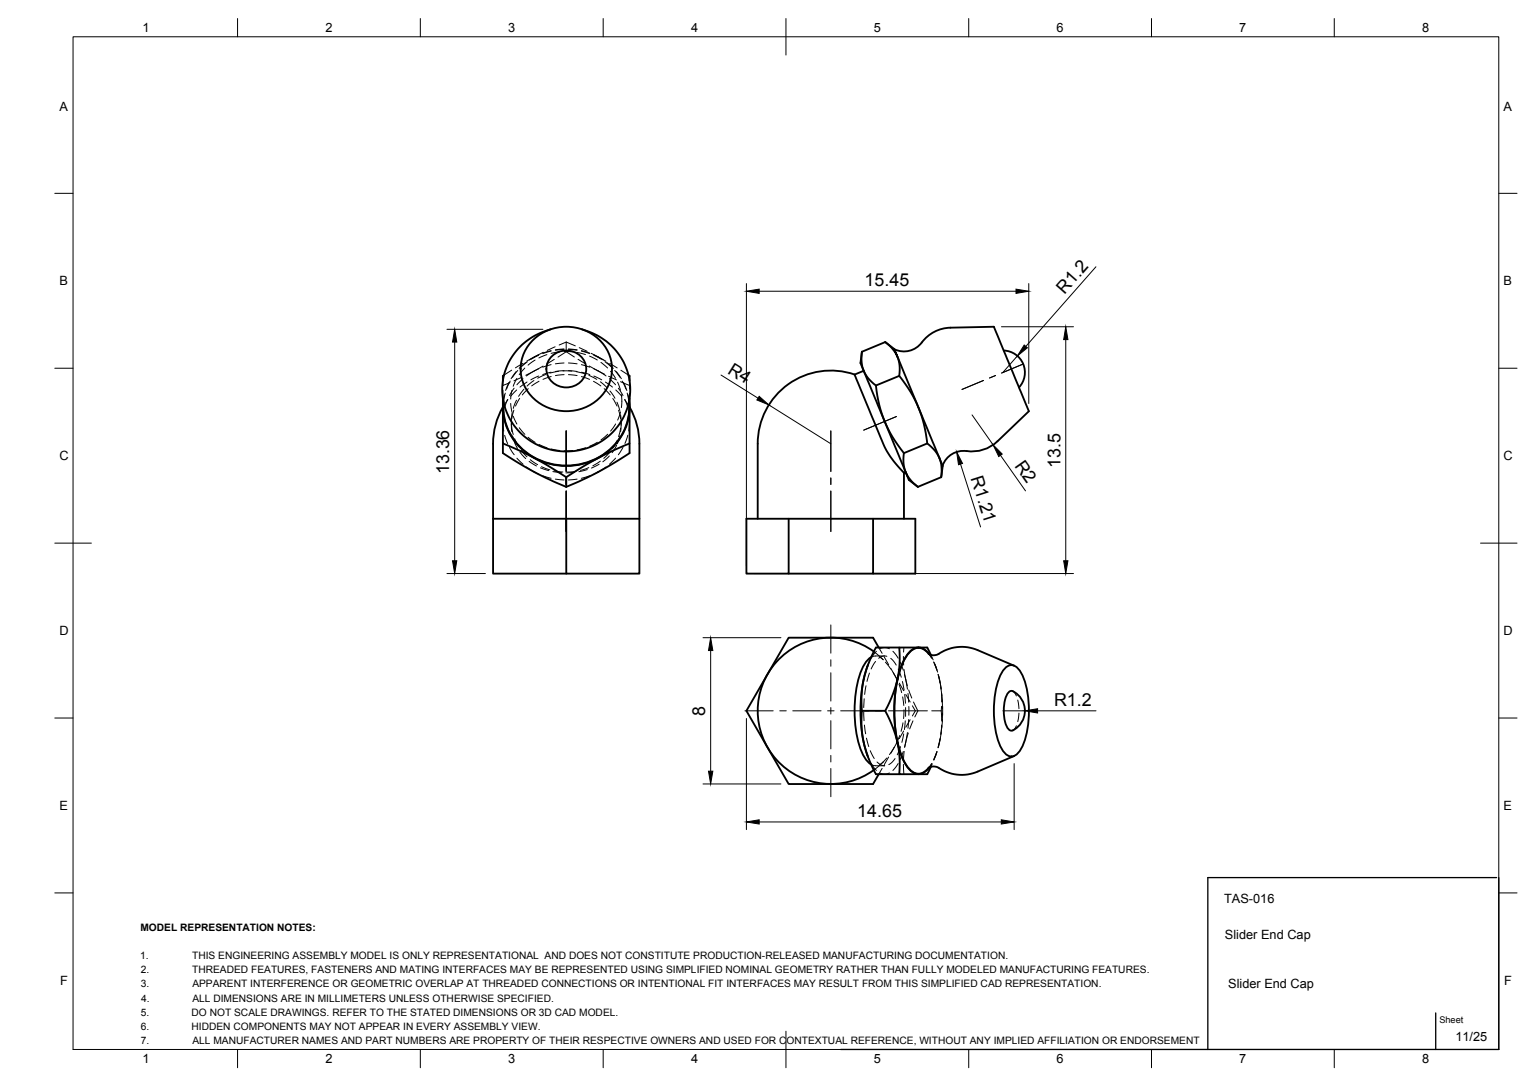
ISO-10303-21;
HEADER;
/* Generated by software containing ST-Developer
 * from STEP Tools, Inc. (www.steptools.com) 
 */

FILE_DESCRIPTION(
/* description */ ('STEP AP214'),
/* implementation_level */ '2;1');

FILE_NAME(
/* name */ 'Slider End Cap.step',
/* time_stamp */ '2026-11-15T14:55:55-08:00',
/* author */ (''),
/* organization */ (''),
/* preprocessor_version */ 'ST-DEVELOPER v20.2',
/* originating_system */ 'Autodesk Translation Framework v15.17.0.0',
/* authorisation */ '');

FILE_SCHEMA (('AUTOMOTIVE_DESIGN { 1 0 10303 214 3 1 1 }'));
ENDSEC;

DATA;
#10=MECHANICAL_DESIGN_GEOMETRIC_PRESENTATION_REPRESENTATION('',(#952),#57079);
#12=(
BOUNDED_CURVE()
B_SPLINE_CURVE(2,(#56108,#56109,#56110),.UNSPECIFIED.,.F.,.F.)
B_SPLINE_CURVE_WITH_KNOTS((3,3),(-1.38994780338837,-1.00314154055664),
 .UNSPECIFIED.)
CURVE()
GEOMETRIC_REPRESENTATION_ITEM()
RATIONAL_B_SPLINE_CURVE((1.79495951130746,1.93380011269289,1.93380011269289))
REPRESENTATION_ITEM('')
);
#13=(
BOUNDED_CURVE()
B_SPLINE_CURVE(2,(#56111,#56112,#56113),.UNSPECIFIED.,.F.,.F.)
B_SPLINE_CURVE_WITH_KNOTS((3,3),(-1.00619430729118,-0.618602381117838),
 .UNSPECIFIED.)
CURVE()
GEOMETRIC_REPRESENTATION_ITEM()
RATIONAL_B_SPLINE_CURVE((1.93745653739061,1.93745653739061,1.7983534165231))
REPRESENTATION_ITEM('')
);
#14=(
BOUNDED_CURVE()
B_SPLINE_CURVE(2,(#56119,#56120,#56121),.UNSPECIFIED.,.F.,.F.)
B_SPLINE_CURVE_WITH_KNOTS((3,3),(-1.38994780338837,-1.00314154055664),
 .UNSPECIFIED.)
CURVE()
GEOMETRIC_REPRESENTATION_ITEM()
RATIONAL_B_SPLINE_CURVE((1.79495951130745,1.93380011269288,1.93380011269288))
REPRESENTATION_ITEM('')
);
#15=(
BOUNDED_CURVE()
B_SPLINE_CURVE(2,(#56122,#56123,#56124),.UNSPECIFIED.,.F.,.F.)
B_SPLINE_CURVE_WITH_KNOTS((3,3),(-1.00619430729117,-0.618602381117832),
 .UNSPECIFIED.)
CURVE()
GEOMETRIC_REPRESENTATION_ITEM()
RATIONAL_B_SPLINE_CURVE((1.9374565373906,1.9374565373906,1.79835341652309))
REPRESENTATION_ITEM('')
);
#16=(
BOUNDED_CURVE()
B_SPLINE_CURVE(2,(#56246,#56247,#56248),.UNSPECIFIED.,.F.,.F.)
B_SPLINE_CURVE_WITH_KNOTS((3,3),(-1.14357963809553,-0.720457873954785),
 .UNSPECIFIED.)
CURVE()
GEOMETRIC_REPRESENTATION_ITEM()
RATIONAL_B_SPLINE_CURVE((2.10284386262275,2.10284386262275,1.95186646604709))
REPRESENTATION_ITEM('')
);
#17=(
BOUNDED_CURVE()
B_SPLINE_CURVE(2,(#56249,#56250,#56251),.UNSPECIFIED.,.F.,.F.)
B_SPLINE_CURVE_WITH_KNOTS((3,3),(-1.51402948258723,-1.10175646251728),
 .UNSPECIFIED.)
CURVE()
GEOMETRIC_REPRESENTATION_ITEM()
RATIONAL_B_SPLINE_CURVE((1.90498640166842,2.0523376126434,2.0523376126434))
REPRESENTATION_ITEM('')
);
#18=(
BOUNDED_CURVE()
B_SPLINE_CURVE(2,(#56254,#56255,#56256),.UNSPECIFIED.,.F.,.F.)
B_SPLINE_CURVE_WITH_KNOTS((3,3),(-1.00619430729147,-0.618602381118052),
 .UNSPECIFIED.)
CURVE()
GEOMETRIC_REPRESENTATION_ITEM()
RATIONAL_B_SPLINE_CURVE((1.93745653739095,1.93745653739095,1.79835341652342))
REPRESENTATION_ITEM('')
);
#19=(
BOUNDED_CURVE()
B_SPLINE_CURVE(2,(#56257,#56258,#56259),.UNSPECIFIED.,.F.,.F.)
B_SPLINE_CURVE_WITH_KNOTS((3,3),(-1.59428966155348,-1.16547770853232),
 .UNSPECIFIED.)
CURVE()
GEOMETRIC_REPRESENTATION_ITEM()
RATIONAL_B_SPLINE_CURVE((1.97645710138757,2.12933659022722,2.12933659022723))
REPRESENTATION_ITEM('')
);
#20=(
BOUNDED_CURVE()
B_SPLINE_CURVE(2,(#56262,#56263,#56264),.UNSPECIFIED.,.F.,.F.)
B_SPLINE_CURVE_WITH_KNOTS((3,3),(-1.39378623346489,-1.00619430729147),
 .UNSPECIFIED.)
CURVE()
GEOMETRIC_REPRESENTATION_ITEM()
RATIONAL_B_SPLINE_CURVE((1.79835341652342,1.93745653739095,1.93745653739095))
REPRESENTATION_ITEM('')
);
#21=(
BOUNDED_CURVE()
B_SPLINE_CURVE(2,(#56265,#56266,#56267),.UNSPECIFIED.,.F.,.F.)
B_SPLINE_CURVE_WITH_KNOTS((3,3),(-1.00314154055692,-0.616335277725119),
 .UNSPECIFIED.)
CURVE()
GEOMETRIC_REPRESENTATION_ITEM()
RATIONAL_B_SPLINE_CURVE((1.93380011269323,1.93380011269323,1.79495951130777))
REPRESENTATION_ITEM('')
);
#22=(
BOUNDED_CURVE()
B_SPLINE_CURVE(2,(#56270,#56271,#56272),.UNSPECIFIED.,.F.,.F.)
B_SPLINE_CURVE_WITH_KNOTS((3,3),(-1.38994780338873,-1.00314154055692),
 .UNSPECIFIED.)
CURVE()
GEOMETRIC_REPRESENTATION_ITEM()
RATIONAL_B_SPLINE_CURVE((1.79495951130777,1.93380011269323,1.93380011269323))
REPRESENTATION_ITEM('')
);
#23=(
BOUNDED_CURVE()
B_SPLINE_CURVE(2,(#56273,#56274,#56275),.UNSPECIFIED.,.F.,.F.)
B_SPLINE_CURVE_WITH_KNOTS((3,3),(-1.16547770853232,-0.73666575551116),
 .UNSPECIFIED.)
CURVE()
GEOMETRIC_REPRESENTATION_ITEM()
RATIONAL_B_SPLINE_CURVE((2.12933659022723,2.12933659022723,1.97645710138758))
REPRESENTATION_ITEM('')
);
#24=(
BOUNDED_CURVE()
B_SPLINE_CURVE(2,(#56278,#56279,#56280),.UNSPECIFIED.,.F.,.F.)
B_SPLINE_CURVE_WITH_KNOTS((3,3),(-1.56670140223628,-1.14357963809553),
 .UNSPECIFIED.)
CURVE()
GEOMETRIC_REPRESENTATION_ITEM()
RATIONAL_B_SPLINE_CURVE((1.95186646604709,2.10284386262275,2.10284386262275))
REPRESENTATION_ITEM('')
);
#25=(
BOUNDED_CURVE()
B_SPLINE_CURVE(2,(#56281,#56282,#56283),.UNSPECIFIED.,.F.,.F.)
B_SPLINE_CURVE_WITH_KNOTS((3,3),(-1.09872453323964,-0.687236958819027),
 .UNSPECIFIED.)
CURVE()
GEOMETRIC_REPRESENTATION_ITEM()
RATIONAL_B_SPLINE_CURVE((2.04868118794568,2.04868118794568,1.90159249645282))
REPRESENTATION_ITEM('')
);
#26=(
BOUNDED_CURVE()
B_SPLINE_CURVE(2,(#56286,#56287,#56288),.UNSPECIFIED.,.F.,.F.)
B_SPLINE_CURVE_WITH_KNOTS((3,3),(-1.56670140224009,-1.14357963809856),
 .UNSPECIFIED.)
CURVE()
GEOMETRIC_REPRESENTATION_ITEM()
RATIONAL_B_SPLINE_CURVE((1.9518664660505,2.10284386262641,2.10284386262641))
REPRESENTATION_ITEM('')
);
#27=(
BOUNDED_CURVE()
B_SPLINE_CURVE(2,(#56289,#56290,#56291),.UNSPECIFIED.,.F.,.F.)
B_SPLINE_CURVE_WITH_KNOTS((3,3),(-1.10777980342349,-0.69394596557458),
 .UNSPECIFIED.)
CURVE()
GEOMETRIC_REPRESENTATION_ITEM()
RATIONAL_B_SPLINE_CURVE((2.05960365436383,2.05960365436383,1.91173076506448))
REPRESENTATION_ITEM('')
);
#28=(
BOUNDED_CURVE()
B_SPLINE_CURVE(2,(#56294,#56295,#56296),.UNSPECIFIED.,.F.,.F.)
B_SPLINE_CURVE_WITH_KNOTS((3,3),(-1.40141169651805,-1.01225852375907),
 .UNSPECIFIED.)
CURVE()
GEOMETRIC_REPRESENTATION_ITEM()
RATIONAL_B_SPLINE_CURVE((1.80509777991977,1.94472257911162,1.94472257911162))
REPRESENTATION_ITEM('')
);
#29=(
BOUNDED_CURVE()
B_SPLINE_CURVE(2,(#56297,#56298,#56299),.UNSPECIFIED.,.F.,.F.)
B_SPLINE_CURVE_WITH_KNOTS((3,3),(-1.16547770853319,-0.736665755511809),
 .UNSPECIFIED.)
CURVE()
GEOMETRIC_REPRESENTATION_ITEM()
RATIONAL_B_SPLINE_CURVE((2.12933659022829,2.12933659022829,1.97645710138856))
REPRESENTATION_ITEM('')
);
#30=(
BOUNDED_CURVE()
B_SPLINE_CURVE(2,(#56302,#56303,#56304),.UNSPECIFIED.,.F.,.F.)
B_SPLINE_CURVE_WITH_KNOTS((3,3),(-1.40141169651807,-1.01225852375909),
 .UNSPECIFIED.)
CURVE()
GEOMETRIC_REPRESENTATION_ITEM()
RATIONAL_B_SPLINE_CURVE((1.80509777991979,1.94472257911164,1.94472257911164))
REPRESENTATION_ITEM('')
);
#31=(
BOUNDED_CURVE()
B_SPLINE_CURVE(2,(#56305,#56306,#56307),.UNSPECIFIED.,.F.,.F.)
B_SPLINE_CURVE_WITH_KNOTS((3,3),(-1.01225852375907,-0.623105351000092),
 .UNSPECIFIED.)
CURVE()
GEOMETRIC_REPRESENTATION_ITEM()
RATIONAL_B_SPLINE_CURVE((1.94472257911162,1.94472257911162,1.80509777991977))
REPRESENTATION_ITEM('')
);
#32=(
BOUNDED_CURVE()
B_SPLINE_CURVE(2,(#56310,#56311,#56312),.UNSPECIFIED.,.F.,.F.)
B_SPLINE_CURVE_WITH_KNOTS((3,3),(-1.59428966155458,-1.16547770853319),
 .UNSPECIFIED.)
CURVE()
GEOMETRIC_REPRESENTATION_ITEM()
RATIONAL_B_SPLINE_CURVE((1.97645710138856,2.12933659022828,2.12933659022828))
REPRESENTATION_ITEM('')
);
#33=(
BOUNDED_CURVE()
B_SPLINE_CURVE(2,(#56313,#56314,#56315),.UNSPECIFIED.,.F.,.F.)
B_SPLINE_CURVE_WITH_KNOTS((3,3),(-1.01225852375909,-0.623105351000104),
 .UNSPECIFIED.)
CURVE()
GEOMETRIC_REPRESENTATION_ITEM()
RATIONAL_B_SPLINE_CURVE((1.94472257911164,1.94472257911164,1.80509777991979))
REPRESENTATION_ITEM('')
);
#34=(
BOUNDED_CURVE()
B_SPLINE_CURVE(2,(#56318,#56319,#56320),.UNSPECIFIED.,.F.,.F.)
B_SPLINE_CURVE_WITH_KNOTS((3,3),(-1.52161364127241,-1.1077798034235),
 .UNSPECIFIED.)
CURVE()
GEOMETRIC_REPRESENTATION_ITEM()
RATIONAL_B_SPLINE_CURVE((1.91173076506449,2.05960365436384,2.05960365436384))
REPRESENTATION_ITEM('')
);
#35=(
BOUNDED_CURVE()
B_SPLINE_CURVE(2,(#56321,#56322,#56323),.UNSPECIFIED.,.F.,.F.)
B_SPLINE_CURVE_WITH_KNOTS((3,3),(-1.14357963809856,-0.720457873957025),
 .UNSPECIFIED.)
CURVE()
GEOMETRIC_REPRESENTATION_ITEM()
RATIONAL_B_SPLINE_CURVE((2.10284386262641,2.10284386262641,1.95186646605049))
REPRESENTATION_ITEM('')
);
#253=(
BOUNDED_SURFACE()
B_SPLINE_SURFACE(2,2,((#56066,#56067,#56068,#56069,#56070,#56071,#56072,
#56073,#56074),(#56075,#56076,#56077,#56078,#56079,#56080,#56081,#56082,
#56083),(#56084,#56085,#56086,#56087,#56088,#56089,#56090,#56091,#56092)),
 .UNSPECIFIED.,.F.,.T.,.F.)
B_SPLINE_SURFACE_WITH_KNOTS((3,3),(3,2,2,2,3),(-0.371257902576148,0.541962924803503),
(-3.14159265358979,-1.5707963267949,0.,1.5707963267949,3.14159265358979),
 .UNSPECIFIED.)
GEOMETRIC_REPRESENTATION_ITEM()
RATIONAL_B_SPLINE_SURFACE(((1.,0.707106781186548,1.,0.707106781186548,1.,
0.707106781186548,1.,0.707106781186548,1.),(0.897552147568833,0.634665210014471,
0.897552147568833,0.634665210014471,0.897552147568833,0.634665210014471,
0.897552147568833,0.634665210014471,0.897552147568833),(1.,0.707106781186548,
1.,0.707106781186548,1.,0.707106781186548,1.,0.707106781186548,1.)))
REPRESENTATION_ITEM('')
SURFACE()
);
#278=SPHERICAL_SURFACE('',#27116,1.2);
#279=SPHERICAL_SURFACE('',#27135,4.);
#648=TOROIDAL_SURFACE('',#27108,4.25,1.21);
#866=B_SPLINE_CURVE_WITH_KNOTS('',3,(#56130,#56131,#56132,#56133,#56134,
#56135,#56136,#56137,#56138,#56139),.UNSPECIFIED.,.F.,.F.,(4,2,2,2,4),(0.112312904835896,
0.113244103065848,0.226488206131697,0.343893756973101,0.461299307814506),
 .UNSPECIFIED.);
#867=B_SPLINE_CURVE_WITH_KNOTS('',3,(#56143,#56144,#56145,#56146,#56147,
#56148,#56149,#56150,#56151,#56152),.UNSPECIFIED.,.F.,.F.,(4,2,2,2,4),(0.461299307814506,
0.57870485865591,0.696110409497315,0.809354512563163,0.810285710793116),
 .UNSPECIFIED.);
#890=SHAPE_REPRESENTATION_RELATIONSHIP('SRR','None',#57280,#919);
#919=ADVANCED_BREP_SHAPE_REPRESENTATION('',(#989),#57072);
#952=STYLED_ITEM('',(#57444),#989);
#989=MANIFOLD_SOLID_BREP('Body1',#24552);
#1315=FACE_BOUND('',#5061,.T.);
#1316=FACE_BOUND('',#5063,.T.);
#1317=FACE_BOUND('',#5094,.T.);
#1999=PLANE('',#27137);
#2000=PLANE('',#27143);
#2001=PLANE('',#27149);
#2002=PLANE('',#27150);
#2003=PLANE('',#27151);
#2004=PLANE('',#27152);
#2005=PLANE('',#27153);
#2006=PLANE('',#27154);
#2007=PLANE('',#27155);
#2008=PLANE('',#27156);
#2009=PLANE('',#27157);
#2010=PLANE('',#27158);
#2011=PLANE('',#27159);
#2012=PLANE('',#27160);
#2013=PLANE('',#27161);
#2014=PLANE('',#27172);
#2015=PLANE('',#27173);
#2016=PLANE('',#27174);
#2017=PLANE('',#27175);
#2018=PLANE('',#27176);
#2019=PLANE('',#27177);
#2020=PLANE('',#27178);
#2128=CONICAL_SURFACE('',#27114,2.5,0.371257902576146);
#2129=CONICAL_SURFACE('',#27118,4.00000000000001,1.04719755119661);
#2130=CONICAL_SURFACE('',#27120,3.46410161513776,1.0471975511966);
#2131=CONICAL_SURFACE('',#27162,3.46410161513776,1.0471975511966);
#2132=CONICAL_SURFACE('',#27163,3.46410161513776,1.0471975511966);
#2133=CONICAL_SURFACE('',#27164,3.46410161513776,1.0471975511966);
#2134=CONICAL_SURFACE('',#27165,3.46410161513776,1.0471975511966);
#2135=CONICAL_SURFACE('',#27166,3.46410161513776,1.0471975511966);
#2136=CONICAL_SURFACE('',#27167,4.00000000000001,1.04719755119661);
#2137=CONICAL_SURFACE('',#27168,4.00000000000001,1.04719755119661);
#2138=CONICAL_SURFACE('',#27169,4.00000000000001,1.04719755119661);
#2139=CONICAL_SURFACE('',#27170,4.00000000000001,1.04719755119661);
#2140=CONICAL_SURFACE('',#27171,4.00000000000001,1.04719755119661);
#3361=FACE_OUTER_BOUND('',#5051,.T.);
#3362=FACE_OUTER_BOUND('',#5052,.T.);
#3363=FACE_OUTER_BOUND('',#5053,.T.);
#3364=FACE_OUTER_BOUND('',#5054,.T.);
#3365=FACE_OUTER_BOUND('',#5055,.T.);
#3366=FACE_OUTER_BOUND('',#5056,.T.);
#3367=FACE_OUTER_BOUND('',#5057,.T.);
#3368=FACE_OUTER_BOUND('',#5058,.T.);
#3369=FACE_OUTER_BOUND('',#5059,.T.);
#3370=FACE_OUTER_BOUND('',#5060,.T.);
#3371=FACE_OUTER_BOUND('',#5062,.T.);
#3372=FACE_OUTER_BOUND('',#5064,.T.);
#3373=FACE_OUTER_BOUND('',#5065,.T.);
#3374=FACE_OUTER_BOUND('',#5066,.T.);
#3375=FACE_OUTER_BOUND('',#5067,.T.);
#3376=FACE_OUTER_BOUND('',#5068,.T.);
#3377=FACE_OUTER_BOUND('',#5069,.T.);
#3378=FACE_OUTER_BOUND('',#5070,.T.);
#3379=FACE_OUTER_BOUND('',#5071,.T.);
#3380=FACE_OUTER_BOUND('',#5072,.T.);
#3381=FACE_OUTER_BOUND('',#5073,.T.);
#3382=FACE_OUTER_BOUND('',#5074,.T.);
#3383=FACE_OUTER_BOUND('',#5075,.T.);
#3384=FACE_OUTER_BOUND('',#5076,.T.);
#3385=FACE_OUTER_BOUND('',#5077,.T.);
#3386=FACE_OUTER_BOUND('',#5078,.T.);
#3387=FACE_OUTER_BOUND('',#5079,.T.);
#3388=FACE_OUTER_BOUND('',#5080,.T.);
#3389=FACE_OUTER_BOUND('',#5081,.T.);
#3390=FACE_OUTER_BOUND('',#5082,.T.);
#3391=FACE_OUTER_BOUND('',#5083,.T.);
#3392=FACE_OUTER_BOUND('',#5084,.T.);
#3393=FACE_OUTER_BOUND('',#5085,.T.);
#3394=FACE_OUTER_BOUND('',#5086,.T.);
#3395=FACE_OUTER_BOUND('',#5087,.T.);
#3396=FACE_OUTER_BOUND('',#5088,.T.);
#3397=FACE_OUTER_BOUND('',#5089,.T.);
#3398=FACE_OUTER_BOUND('',#5090,.T.);
#3399=FACE_OUTER_BOUND('',#5091,.T.);
#3400=FACE_OUTER_BOUND('',#5092,.T.);
#3401=FACE_OUTER_BOUND('',#5093,.T.);
#5051=EDGE_LOOP('',(#22016,#22017,#22018,#22019));
#5052=EDGE_LOOP('',(#22020,#22021,#22022,#22023));
#5053=EDGE_LOOP('',(#22024,#22025,#22026,#22027));
#5054=EDGE_LOOP('',(#22028));
#5055=EDGE_LOOP('',(#22029,#22030,#22031));
#5056=EDGE_LOOP('',(#22032,#22033,#22034));
#5057=EDGE_LOOP('',(#22035,#22036,#22037,#22038,#22039,#22040));
#5058=EDGE_LOOP('',(#22041,#22042,#22043,#22044,#22045,#22046,#22047,#22048,
#22049,#22050,#22051,#22052,#22053));
#5059=EDGE_LOOP('',(#22054,#22055,#22056,#22057,#22058,#22059));
#5060=EDGE_LOOP('',(#22060,#22061,#22062,#22063,#22064,#22065));
#5061=EDGE_LOOP('',(#22066));
#5062=EDGE_LOOP('',(#22067,#22068,#22069,#22070,#22071,#22072));
#5063=EDGE_LOOP('',(#22073));
#5064=EDGE_LOOP('',(#22074,#22075,#22076));
#5065=EDGE_LOOP('',(#22077,#22078,#22079));
#5066=EDGE_LOOP('',(#22080,#22081,#22082));
#5067=EDGE_LOOP('',(#22083,#22084,#22085));
#5068=EDGE_LOOP('',(#22086,#22087,#22088));
#5069=EDGE_LOOP('',(#22089,#22090,#22091));
#5070=EDGE_LOOP('',(#22092,#22093,#22094,#22095,#22096));
#5071=EDGE_LOOP('',(#22097,#22098,#22099,#22100,#22101));
#5072=EDGE_LOOP('',(#22102,#22103,#22104,#22105,#22106));
#5073=EDGE_LOOP('',(#22107,#22108,#22109,#22110,#22111));
#5074=EDGE_LOOP('',(#22112,#22113,#22114,#22115,#22116));
#5075=EDGE_LOOP('',(#22117,#22118,#22119,#22120,#22121));
#5076=EDGE_LOOP('',(#22122,#22123,#22124,#22125,#22126,#22127));
#5077=EDGE_LOOP('',(#22128,#22129,#22130));
#5078=EDGE_LOOP('',(#22131,#22132,#22133));
#5079=EDGE_LOOP('',(#22134,#22135,#22136));
#5080=EDGE_LOOP('',(#22137,#22138,#22139));
#5081=EDGE_LOOP('',(#22140,#22141,#22142));
#5082=EDGE_LOOP('',(#22143,#22144,#22145));
#5083=EDGE_LOOP('',(#22146,#22147,#22148));
#5084=EDGE_LOOP('',(#22149,#22150,#22151));
#5085=EDGE_LOOP('',(#22152,#22153,#22154));
#5086=EDGE_LOOP('',(#22155,#22156,#22157));
#5087=EDGE_LOOP('',(#22158,#22159,#22160,#22161,#22162,#22163));
#5088=EDGE_LOOP('',(#22164,#22165,#22166,#22167,#22168,#22169));
#5089=EDGE_LOOP('',(#22170,#22171,#22172,#22173,#22174,#22175));
#5090=EDGE_LOOP('',(#22176,#22177,#22178,#22179,#22180,#22181));
#5091=EDGE_LOOP('',(#22182,#22183,#22184,#22185,#22186,#22187));
#5092=EDGE_LOOP('',(#22188,#22189,#22190,#22191,#22192,#22193));
#5093=EDGE_LOOP('',(#22194));
#5094=EDGE_LOOP('',(#22195));
#6999=LINE('',#56098,#8966);
#7000=LINE('',#56141,#8967);
#7001=LINE('',#56160,#8968);
#7002=LINE('',#56197,#8969);
#7003=LINE('',#56198,#8970);
#7004=LINE('',#56201,#8971);
#7005=LINE('',#56202,#8972);
#7006=LINE('',#56205,#8973);
#7007=LINE('',#56206,#8974);
#7008=LINE('',#56209,#8975);
#7009=LINE('',#56210,#8976);
#7010=LINE('',#56213,#8977);
#7011=LINE('',#56214,#8978);
#7012=LINE('',#56217,#8979);
#7013=LINE('',#56218,#8980);
#7014=LINE('',#56222,#8981);
#7015=LINE('',#56223,#8982);
#7016=LINE('',#56224,#8983);
#7017=LINE('',#56227,#8984);
#7018=LINE('',#56228,#8985);
#7019=LINE('',#56231,#8986);
#7020=LINE('',#56232,#8987);
#7021=LINE('',#56235,#8988);
#7022=LINE('',#56236,#8989);
#7023=LINE('',#56239,#8990);
#7024=LINE('',#56240,#8991);
#7025=LINE('',#56242,#8992);
#7026=LINE('',#56325,#8993);
#7027=LINE('',#56326,#8994);
#7028=LINE('',#56328,#8995);
#7029=LINE('',#56330,#8996);
#7030=LINE('',#56332,#8997);
#7031=LINE('',#56334,#8998);
#8966=VECTOR('',#33689,2.5);
#8967=VECTOR('',#33708,3.);
#8968=VECTOR('',#33719,4.);
#8969=VECTOR('',#33762,1000.);
#8970=VECTOR('',#33763,1000.);
#8971=VECTOR('',#33766,1000.);
#8972=VECTOR('',#33767,1000.);
#8973=VECTOR('',#33770,1000.);
#8974=VECTOR('',#33771,1000.);
#8975=VECTOR('',#33774,1000.);
#8976=VECTOR('',#33775,1000.);
#8977=VECTOR('',#33778,1000.);
#8978=VECTOR('',#33779,1000.);
#8979=VECTOR('',#33782,1000.);
#8980=VECTOR('',#33783,1000.);
#8981=VECTOR('',#33786,1000.);
#8982=VECTOR('',#33787,1000.);
#8983=VECTOR('',#33788,1000.);
#8984=VECTOR('',#33791,1000.);
#8985=VECTOR('',#33792,1000.);
#8986=VECTOR('',#33795,1000.);
#8987=VECTOR('',#33796,1000.);
#8988=VECTOR('',#33799,1000.);
#8989=VECTOR('',#33800,1000.);
#8990=VECTOR('',#33803,1000.);
#8991=VECTOR('',#33804,1000.);
#8992=VECTOR('',#33807,1000.);
#8993=VECTOR('',#33832,1000.);
#8994=VECTOR('',#33833,1000.);
#8995=VECTOR('',#33836,1000.);
#8996=VECTOR('',#33839,1000.);
#8997=VECTOR('',#33842,1000.);
#8998=VECTOR('',#33845,1000.);
#10161=CIRCLE('',#27109,3.44123551017618);
#10162=CIRCLE('',#27110,1.21);
#10163=CIRCLE('',#27111,3.21339563862929);
#10164=CIRCLE('',#27112,2.);
#10165=CIRCLE('',#27113,3.36374346224613);
#10166=CIRCLE('',#27115,2.5);
#10167=CIRCLE('',#27117,1.09087121146357);
#10168=CIRCLE('',#27119,3.46410161513777);
#10169=CIRCLE('',#27121,3.46410161513775);
#10170=CIRCLE('',#27123,3.);
#10171=CIRCLE('',#27124,3.);
#10172=CIRCLE('',#27126,4.);
#10173=CIRCLE('',#27127,4.);
#10174=CIRCLE('',#27128,4.);
#10175=CIRCLE('',#27129,4.);
#10176=CIRCLE('',#27130,4.);
#10177=CIRCLE('',#27131,4.);
#10178=CIRCLE('',#27132,4.);
#10179=CIRCLE('',#27133,4.);
#10180=CIRCLE('',#27134,4.);
#10181=CIRCLE('',#27136,4.);
#10182=CIRCLE('',#27138,3.46410161513776);
#10183=CIRCLE('',#27139,3.46410161513777);
#10184=CIRCLE('',#27140,3.46410161513777);
#10185=CIRCLE('',#27141,3.46410161513777);
#10186=CIRCLE('',#27142,3.46410161513777);
#10187=CIRCLE('',#27144,3.46410161513775);
#10188=CIRCLE('',#27145,3.46410161513775);
#10189=CIRCLE('',#27146,3.46410161513775);
#10190=CIRCLE('',#27147,3.46410161513775);
#10191=CIRCLE('',#27148,3.46410161513776);
#12268=VERTEX_POINT('',#56061);
#12269=VERTEX_POINT('',#56063);
#12270=VERTEX_POINT('',#56093);
#12271=VERTEX_POINT('',#56097);
#12272=VERTEX_POINT('',#56101);
#12273=VERTEX_POINT('',#56104);
#12274=VERTEX_POINT('',#56105);
#12275=VERTEX_POINT('',#56107);
#12276=VERTEX_POINT('',#56115);
#12277=VERTEX_POINT('',#56116);
#12278=VERTEX_POINT('',#56118);
#12279=VERTEX_POINT('',#56126);
#12280=VERTEX_POINT('',#56127);
#12281=VERTEX_POINT('',#56129);
#12282=VERTEX_POINT('',#56140);
#12283=VERTEX_POINT('',#56154);
#12284=VERTEX_POINT('',#56156);
#12285=VERTEX_POINT('',#56159);
#12286=VERTEX_POINT('',#56161);
#12287=VERTEX_POINT('',#56163);
#12288=VERTEX_POINT('',#56165);
#12289=VERTEX_POINT('',#56167);
#12290=VERTEX_POINT('',#56169);
#12291=VERTEX_POINT('',#56173);
#12292=VERTEX_POINT('',#56176);
#12293=VERTEX_POINT('',#56178);
#12294=VERTEX_POINT('',#56180);
#12295=VERTEX_POINT('',#56182);
#12296=VERTEX_POINT('',#56186);
#12297=VERTEX_POINT('',#56188);
#12298=VERTEX_POINT('',#56190);
#12299=VERTEX_POINT('',#56192);
#12300=VERTEX_POINT('',#56196);
#12301=VERTEX_POINT('',#56200);
#12302=VERTEX_POINT('',#56204);
#12303=VERTEX_POINT('',#56208);
#12304=VERTEX_POINT('',#56212);
#12305=VERTEX_POINT('',#56216);
#12306=VERTEX_POINT('',#56220);
#12307=VERTEX_POINT('',#56221);
#12308=VERTEX_POINT('',#56226);
#12309=VERTEX_POINT('',#56230);
#12310=VERTEX_POINT('',#56234);
#12311=VERTEX_POINT('',#56238);
#12312=VERTEX_POINT('',#56245);
#12313=VERTEX_POINT('',#56253);
#12314=VERTEX_POINT('',#56261);
#12315=VERTEX_POINT('',#56269);
#12316=VERTEX_POINT('',#56277);
#12317=VERTEX_POINT('',#56285);
#12318=VERTEX_POINT('',#56293);
#12319=VERTEX_POINT('',#56301);
#12320=VERTEX_POINT('',#56309);
#12321=VERTEX_POINT('',#56317);
#15553=EDGE_CURVE('',#12268,#12268,#10161,.T.);
#15554=EDGE_CURVE('',#12268,#12269,#10162,.T.);
#15555=EDGE_CURVE('',#12269,#12269,#10163,.T.);
#15556=EDGE_CURVE('',#12269,#12270,#10164,.T.);
#15557=EDGE_CURVE('',#12270,#12270,#10165,.T.);
#15558=EDGE_CURVE('',#12270,#12271,#6999,.T.);
#15559=EDGE_CURVE('',#12271,#12271,#10166,.T.);
#15560=EDGE_CURVE('',#12272,#12272,#10167,.T.);
#15561=EDGE_CURVE('',#12273,#12274,#10168,.T.);
#15562=EDGE_CURVE('',#12275,#12274,#12,.T.);
#15563=EDGE_CURVE('',#12273,#12275,#13,.T.);
#15564=EDGE_CURVE('',#12276,#12277,#10169,.T.);
#15565=EDGE_CURVE('',#12278,#12277,#14,.T.);
#15566=EDGE_CURVE('',#12276,#12278,#15,.T.);
#15567=EDGE_CURVE('',#12279,#12280,#10170,.T.);
#15568=EDGE_CURVE('',#12281,#12279,#866,.F.);
#15569=EDGE_CURVE('',#12281,#12282,#7000,.T.);
#15570=EDGE_CURVE('',#12282,#12282,#10171,.T.);
#15571=EDGE_CURVE('',#12280,#12281,#867,.F.);
#15572=EDGE_CURVE('',#12280,#12283,#10172,.T.);
#15573=EDGE_CURVE('',#12284,#12279,#10173,.T.);
#15574=EDGE_CURVE('',#12283,#12284,#10174,.T.);
#15575=EDGE_CURVE('',#12283,#12285,#7001,.T.);
#15576=EDGE_CURVE('',#12285,#12286,#10175,.T.);
#15577=EDGE_CURVE('',#12286,#12287,#10176,.T.);
#15578=EDGE_CURVE('',#12287,#12288,#10177,.T.);
#15579=EDGE_CURVE('',#12288,#12289,#10178,.T.);
#15580=EDGE_CURVE('',#12289,#12290,#10179,.T.);
#15581=EDGE_CURVE('',#12290,#12285,#10180,.T.);
#15582=EDGE_CURVE('',#12284,#12291,#10181,.T.);
#15583=EDGE_CURVE('',#12274,#12292,#10182,.T.);
#15584=EDGE_CURVE('',#12293,#12273,#10183,.T.);
#15585=EDGE_CURVE('',#12294,#12293,#10184,.T.);
#15586=EDGE_CURVE('',#12295,#12294,#10185,.T.);
#15587=EDGE_CURVE('',#12292,#12295,#10186,.T.);
#15588=EDGE_CURVE('',#12277,#12296,#10187,.T.);
#15589=EDGE_CURVE('',#12297,#12276,#10188,.T.);
#15590=EDGE_CURVE('',#12298,#12297,#10189,.T.);
#15591=EDGE_CURVE('',#12299,#12298,#10190,.T.);
#15592=EDGE_CURVE('',#12299,#12296,#10191,.T.);
#15593=EDGE_CURVE('',#12300,#12288,#7002,.T.);
#15594=EDGE_CURVE('',#12289,#12300,#7003,.T.);
#15595=EDGE_CURVE('',#12301,#12289,#7004,.T.);
#15596=EDGE_CURVE('',#12290,#12301,#7005,.T.);
#15597=EDGE_CURVE('',#12302,#12290,#7006,.T.);
#15598=EDGE_CURVE('',#12285,#12302,#7007,.T.);
#15599=EDGE_CURVE('',#12303,#12285,#7008,.T.);
#15600=EDGE_CURVE('',#12286,#12303,#7009,.T.);
#15601=EDGE_CURVE('',#12304,#12286,#7010,.T.);
#15602=EDGE_CURVE('',#12287,#12304,#7011,.T.);
#15603=EDGE_CURVE('',#12305,#12287,#7012,.T.);
#15604=EDGE_CURVE('',#12288,#12305,#7013,.T.);
#15605=EDGE_CURVE('',#12306,#12307,#7014,.T.);
#15606=EDGE_CURVE('',#12302,#12306,#7015,.T.);
#15607=EDGE_CURVE('',#12301,#12307,#7016,.T.);
#15608=EDGE_CURVE('',#12308,#12306,#7017,.T.);
#15609=EDGE_CURVE('',#12303,#12308,#7018,.T.);
#15610=EDGE_CURVE('',#12309,#12308,#7019,.T.);
#15611=EDGE_CURVE('',#12304,#12309,#7020,.T.);
#15612=EDGE_CURVE('',#12310,#12309,#7021,.T.);
#15613=EDGE_CURVE('',#12305,#12310,#7022,.T.);
#15614=EDGE_CURVE('',#12311,#12310,#7023,.T.);
#15615=EDGE_CURVE('',#12300,#12311,#7024,.T.);
#15616=EDGE_CURVE('',#12307,#12311,#7025,.T.);
#15617=EDGE_CURVE('',#12297,#12312,#16,.T.);
#15618=EDGE_CURVE('',#12312,#12276,#17,.T.);
#15619=EDGE_CURVE('',#12298,#12313,#18,.T.);
#15620=EDGE_CURVE('',#12313,#12297,#19,.T.);
#15621=EDGE_CURVE('',#12314,#12298,#20,.T.);
#15622=EDGE_CURVE('',#12299,#12314,#21,.T.);
#15623=EDGE_CURVE('',#12315,#12299,#22,.T.);
#15624=EDGE_CURVE('',#12296,#12315,#23,.T.);
#15625=EDGE_CURVE('',#12316,#12296,#24,.T.);
#15626=EDGE_CURVE('',#12277,#12316,#25,.T.);
#15627=EDGE_CURVE('',#12317,#12292,#26,.T.);
#15628=EDGE_CURVE('',#12274,#12317,#27,.T.);
#15629=EDGE_CURVE('',#12318,#12295,#28,.T.);
#15630=EDGE_CURVE('',#12292,#12318,#29,.T.);
#15631=EDGE_CURVE('',#12319,#12294,#30,.T.);
#15632=EDGE_CURVE('',#12295,#12319,#31,.T.);
#15633=EDGE_CURVE('',#12320,#12293,#32,.T.);
#15634=EDGE_CURVE('',#12294,#12320,#33,.T.);
#15635=EDGE_CURVE('',#12321,#12273,#34,.T.);
#15636=EDGE_CURVE('',#12293,#12321,#35,.T.);
#15637=EDGE_CURVE('',#12314,#12275,#7026,.T.);
#15638=EDGE_CURVE('',#12313,#12321,#7027,.T.);
#15639=EDGE_CURVE('',#12312,#12320,#7028,.T.);
#15640=EDGE_CURVE('',#12278,#12319,#7029,.T.);
#15641=EDGE_CURVE('',#12316,#12318,#7030,.T.);
#15642=EDGE_CURVE('',#12315,#12317,#7031,.T.);
#22016=ORIENTED_EDGE('',*,*,#15553,.T.);
#22017=ORIENTED_EDGE('',*,*,#15554,.T.);
#22018=ORIENTED_EDGE('',*,*,#15555,.T.);
#22019=ORIENTED_EDGE('',*,*,#15554,.F.);
#22020=ORIENTED_EDGE('',*,*,#15555,.F.);
#22021=ORIENTED_EDGE('',*,*,#15556,.T.);
#22022=ORIENTED_EDGE('',*,*,#15557,.T.);
#22023=ORIENTED_EDGE('',*,*,#15556,.F.);
#22024=ORIENTED_EDGE('',*,*,#15557,.F.);
#22025=ORIENTED_EDGE('',*,*,#15558,.T.);
#22026=ORIENTED_EDGE('',*,*,#15559,.T.);
#22027=ORIENTED_EDGE('',*,*,#15558,.F.);
#22028=ORIENTED_EDGE('',*,*,#15560,.F.);
#22029=ORIENTED_EDGE('',*,*,#15561,.T.);
#22030=ORIENTED_EDGE('',*,*,#15562,.F.);
#22031=ORIENTED_EDGE('',*,*,#15563,.F.);
#22032=ORIENTED_EDGE('',*,*,#15564,.T.);
#22033=ORIENTED_EDGE('',*,*,#15565,.F.);
#22034=ORIENTED_EDGE('',*,*,#15566,.F.);
#22035=ORIENTED_EDGE('',*,*,#15567,.F.);
#22036=ORIENTED_EDGE('',*,*,#15568,.F.);
#22037=ORIENTED_EDGE('',*,*,#15569,.T.);
#22038=ORIENTED_EDGE('',*,*,#15570,.T.);
#22039=ORIENTED_EDGE('',*,*,#15569,.F.);
#22040=ORIENTED_EDGE('',*,*,#15571,.F.);
#22041=ORIENTED_EDGE('',*,*,#15572,.F.);
#22042=ORIENTED_EDGE('',*,*,#15571,.T.);
#22043=ORIENTED_EDGE('',*,*,#15568,.T.);
#22044=ORIENTED_EDGE('',*,*,#15573,.F.);
#22045=ORIENTED_EDGE('',*,*,#15574,.F.);
#22046=ORIENTED_EDGE('',*,*,#15575,.T.);
#22047=ORIENTED_EDGE('',*,*,#15576,.T.);
#22048=ORIENTED_EDGE('',*,*,#15577,.T.);
#22049=ORIENTED_EDGE('',*,*,#15578,.T.);
#22050=ORIENTED_EDGE('',*,*,#15579,.T.);
#22051=ORIENTED_EDGE('',*,*,#15580,.T.);
#22052=ORIENTED_EDGE('',*,*,#15581,.T.);
#22053=ORIENTED_EDGE('',*,*,#15575,.F.);
#22054=ORIENTED_EDGE('',*,*,#15572,.T.);
#22055=ORIENTED_EDGE('',*,*,#15574,.T.);
#22056=ORIENTED_EDGE('',*,*,#15582,.T.);
#22057=ORIENTED_EDGE('',*,*,#15582,.F.);
#22058=ORIENTED_EDGE('',*,*,#15573,.T.);
#22059=ORIENTED_EDGE('',*,*,#15567,.T.);
#22060=ORIENTED_EDGE('',*,*,#15583,.F.);
#22061=ORIENTED_EDGE('',*,*,#15561,.F.);
#22062=ORIENTED_EDGE('',*,*,#15584,.F.);
#22063=ORIENTED_EDGE('',*,*,#15585,.F.);
#22064=ORIENTED_EDGE('',*,*,#15586,.F.);
#22065=ORIENTED_EDGE('',*,*,#15587,.F.);
#22066=ORIENTED_EDGE('',*,*,#15553,.F.);
#22067=ORIENTED_EDGE('',*,*,#15588,.F.);
#22068=ORIENTED_EDGE('',*,*,#15564,.F.);
#22069=ORIENTED_EDGE('',*,*,#15589,.F.);
#22070=ORIENTED_EDGE('',*,*,#15590,.F.);
#22071=ORIENTED_EDGE('',*,*,#15591,.F.);
#22072=ORIENTED_EDGE('',*,*,#15592,.T.);
#22073=ORIENTED_EDGE('',*,*,#15570,.F.);
#22074=ORIENTED_EDGE('',*,*,#15579,.F.);
#22075=ORIENTED_EDGE('',*,*,#15593,.F.);
#22076=ORIENTED_EDGE('',*,*,#15594,.F.);
#22077=ORIENTED_EDGE('',*,*,#15580,.F.);
#22078=ORIENTED_EDGE('',*,*,#15595,.F.);
#22079=ORIENTED_EDGE('',*,*,#15596,.F.);
#22080=ORIENTED_EDGE('',*,*,#15581,.F.);
#22081=ORIENTED_EDGE('',*,*,#15597,.F.);
#22082=ORIENTED_EDGE('',*,*,#15598,.F.);
#22083=ORIENTED_EDGE('',*,*,#15576,.F.);
#22084=ORIENTED_EDGE('',*,*,#15599,.F.);
#22085=ORIENTED_EDGE('',*,*,#15600,.F.);
#22086=ORIENTED_EDGE('',*,*,#15577,.F.);
#22087=ORIENTED_EDGE('',*,*,#15601,.F.);
#22088=ORIENTED_EDGE('',*,*,#15602,.F.);
#22089=ORIENTED_EDGE('',*,*,#15578,.F.);
#22090=ORIENTED_EDGE('',*,*,#15603,.F.);
#22091=ORIENTED_EDGE('',*,*,#15604,.F.);
#22092=ORIENTED_EDGE('',*,*,#15605,.F.);
#22093=ORIENTED_EDGE('',*,*,#15606,.F.);
#22094=ORIENTED_EDGE('',*,*,#15597,.T.);
#22095=ORIENTED_EDGE('',*,*,#15596,.T.);
#22096=ORIENTED_EDGE('',*,*,#15607,.T.);
#22097=ORIENTED_EDGE('',*,*,#15608,.F.);
#22098=ORIENTED_EDGE('',*,*,#15609,.F.);
#22099=ORIENTED_EDGE('',*,*,#15599,.T.);
#22100=ORIENTED_EDGE('',*,*,#15598,.T.);
#22101=ORIENTED_EDGE('',*,*,#15606,.T.);
#22102=ORIENTED_EDGE('',*,*,#15610,.F.);
#22103=ORIENTED_EDGE('',*,*,#15611,.F.);
#22104=ORIENTED_EDGE('',*,*,#15601,.T.);
#22105=ORIENTED_EDGE('',*,*,#15600,.T.);
#22106=ORIENTED_EDGE('',*,*,#15609,.T.);
#22107=ORIENTED_EDGE('',*,*,#15612,.F.);
#22108=ORIENTED_EDGE('',*,*,#15613,.F.);
#22109=ORIENTED_EDGE('',*,*,#15603,.T.);
#22110=ORIENTED_EDGE('',*,*,#15602,.T.);
#22111=ORIENTED_EDGE('',*,*,#15611,.T.);
#22112=ORIENTED_EDGE('',*,*,#15614,.F.);
#22113=ORIENTED_EDGE('',*,*,#15615,.F.);
#22114=ORIENTED_EDGE('',*,*,#15593,.T.);
#22115=ORIENTED_EDGE('',*,*,#15604,.T.);
#22116=ORIENTED_EDGE('',*,*,#15613,.T.);
#22117=ORIENTED_EDGE('',*,*,#15616,.F.);
#22118=ORIENTED_EDGE('',*,*,#15607,.F.);
#22119=ORIENTED_EDGE('',*,*,#15595,.T.);
#22120=ORIENTED_EDGE('',*,*,#15594,.T.);
#22121=ORIENTED_EDGE('',*,*,#15615,.T.);
#22122=ORIENTED_EDGE('',*,*,#15605,.T.);
#22123=ORIENTED_EDGE('',*,*,#15616,.T.);
#22124=ORIENTED_EDGE('',*,*,#15614,.T.);
#22125=ORIENTED_EDGE('',*,*,#15612,.T.);
#22126=ORIENTED_EDGE('',*,*,#15610,.T.);
#22127=ORIENTED_EDGE('',*,*,#15608,.T.);
#22128=ORIENTED_EDGE('',*,*,#15617,.F.);
#22129=ORIENTED_EDGE('',*,*,#15589,.T.);
#22130=ORIENTED_EDGE('',*,*,#15618,.F.);
#22131=ORIENTED_EDGE('',*,*,#15619,.F.);
#22132=ORIENTED_EDGE('',*,*,#15590,.T.);
#22133=ORIENTED_EDGE('',*,*,#15620,.F.);
#22134=ORIENTED_EDGE('',*,*,#15591,.T.);
#22135=ORIENTED_EDGE('',*,*,#15621,.F.);
#22136=ORIENTED_EDGE('',*,*,#15622,.F.);
#22137=ORIENTED_EDGE('',*,*,#15592,.F.);
#22138=ORIENTED_EDGE('',*,*,#15623,.F.);
#22139=ORIENTED_EDGE('',*,*,#15624,.F.);
#22140=ORIENTED_EDGE('',*,*,#15588,.T.);
#22141=ORIENTED_EDGE('',*,*,#15625,.F.);
#22142=ORIENTED_EDGE('',*,*,#15626,.F.);
#22143=ORIENTED_EDGE('',*,*,#15583,.T.);
#22144=ORIENTED_EDGE('',*,*,#15627,.F.);
#22145=ORIENTED_EDGE('',*,*,#15628,.F.);
#22146=ORIENTED_EDGE('',*,*,#15587,.T.);
#22147=ORIENTED_EDGE('',*,*,#15629,.F.);
#22148=ORIENTED_EDGE('',*,*,#15630,.F.);
#22149=ORIENTED_EDGE('',*,*,#15586,.T.);
#22150=ORIENTED_EDGE('',*,*,#15631,.F.);
#22151=ORIENTED_EDGE('',*,*,#15632,.F.);
#22152=ORIENTED_EDGE('',*,*,#15585,.T.);
#22153=ORIENTED_EDGE('',*,*,#15633,.F.);
#22154=ORIENTED_EDGE('',*,*,#15634,.F.);
#22155=ORIENTED_EDGE('',*,*,#15584,.T.);
#22156=ORIENTED_EDGE('',*,*,#15635,.F.);
#22157=ORIENTED_EDGE('',*,*,#15636,.F.);
#22158=ORIENTED_EDGE('',*,*,#15637,.F.);
#22159=ORIENTED_EDGE('',*,*,#15621,.T.);
#22160=ORIENTED_EDGE('',*,*,#15619,.T.);
#22161=ORIENTED_EDGE('',*,*,#15638,.T.);
#22162=ORIENTED_EDGE('',*,*,#15635,.T.);
#22163=ORIENTED_EDGE('',*,*,#15563,.T.);
#22164=ORIENTED_EDGE('',*,*,#15638,.F.);
#22165=ORIENTED_EDGE('',*,*,#15620,.T.);
#22166=ORIENTED_EDGE('',*,*,#15617,.T.);
#22167=ORIENTED_EDGE('',*,*,#15639,.T.);
#22168=ORIENTED_EDGE('',*,*,#15633,.T.);
#22169=ORIENTED_EDGE('',*,*,#15636,.T.);
#22170=ORIENTED_EDGE('',*,*,#15639,.F.);
#22171=ORIENTED_EDGE('',*,*,#15618,.T.);
#22172=ORIENTED_EDGE('',*,*,#15566,.T.);
#22173=ORIENTED_EDGE('',*,*,#15640,.T.);
#22174=ORIENTED_EDGE('',*,*,#15631,.T.);
#22175=ORIENTED_EDGE('',*,*,#15634,.T.);
#22176=ORIENTED_EDGE('',*,*,#15640,.F.);
#22177=ORIENTED_EDGE('',*,*,#15565,.T.);
#22178=ORIENTED_EDGE('',*,*,#15626,.T.);
#22179=ORIENTED_EDGE('',*,*,#15641,.T.);
#22180=ORIENTED_EDGE('',*,*,#15629,.T.);
#22181=ORIENTED_EDGE('',*,*,#15632,.T.);
#22182=ORIENTED_EDGE('',*,*,#15641,.F.);
#22183=ORIENTED_EDGE('',*,*,#15625,.T.);
#22184=ORIENTED_EDGE('',*,*,#15624,.T.);
#22185=ORIENTED_EDGE('',*,*,#15642,.T.);
#22186=ORIENTED_EDGE('',*,*,#15627,.T.);
#22187=ORIENTED_EDGE('',*,*,#15630,.T.);
#22188=ORIENTED_EDGE('',*,*,#15642,.F.);
#22189=ORIENTED_EDGE('',*,*,#15623,.T.);
#22190=ORIENTED_EDGE('',*,*,#15622,.T.);
#22191=ORIENTED_EDGE('',*,*,#15637,.T.);
#22192=ORIENTED_EDGE('',*,*,#15562,.T.);
#22193=ORIENTED_EDGE('',*,*,#15628,.T.);
#22194=ORIENTED_EDGE('',*,*,#15559,.F.);
#22195=ORIENTED_EDGE('',*,*,#15560,.T.);
#23119=CYLINDRICAL_SURFACE('',#27122,3.);
#23120=CYLINDRICAL_SURFACE('',#27125,4.);
#24353=ADVANCED_FACE('',(#3361),#648,.F.);
#24354=ADVANCED_FACE('',(#3362),#253,.F.);
#24355=ADVANCED_FACE('',(#3363),#2128,.T.);
#24356=ADVANCED_FACE('',(#3364),#278,.T.);
#24357=ADVANCED_FACE('',(#3365),#2129,.T.);
#24358=ADVANCED_FACE('',(#3366),#2130,.T.);
#24359=ADVANCED_FACE('',(#3367),#23119,.T.);
#24360=ADVANCED_FACE('',(#3368),#23120,.T.);
#24361=ADVANCED_FACE('',(#3369),#279,.T.);
#24362=ADVANCED_FACE('',(#3370,#1315),#1999,.F.);
#24363=ADVANCED_FACE('',(#3371,#1316),#2000,.F.);
#24364=ADVANCED_FACE('',(#3372),#2001,.F.);
#24365=ADVANCED_FACE('',(#3373),#2002,.F.);
#24366=ADVANCED_FACE('',(#3374),#2003,.F.);
#24367=ADVANCED_FACE('',(#3375),#2004,.F.);
#24368=ADVANCED_FACE('',(#3376),#2005,.F.);
#24369=ADVANCED_FACE('',(#3377),#2006,.F.);
#24370=ADVANCED_FACE('',(#3378),#2007,.T.);
#24371=ADVANCED_FACE('',(#3379),#2008,.T.);
#24372=ADVANCED_FACE('',(#3380),#2009,.T.);
#24373=ADVANCED_FACE('',(#3381),#2010,.T.);
#24374=ADVANCED_FACE('',(#3382),#2011,.T.);
#24375=ADVANCED_FACE('',(#3383),#2012,.T.);
#24376=ADVANCED_FACE('',(#3384),#2013,.T.);
#24377=ADVANCED_FACE('',(#3385),#2131,.T.);
#24378=ADVANCED_FACE('',(#3386),#2132,.T.);
#24379=ADVANCED_FACE('',(#3387),#2133,.T.);
#24380=ADVANCED_FACE('',(#3388),#2134,.T.);
#24381=ADVANCED_FACE('',(#3389),#2135,.T.);
#24382=ADVANCED_FACE('',(#3390),#2136,.T.);
#24383=ADVANCED_FACE('',(#3391),#2137,.T.);
#24384=ADVANCED_FACE('',(#3392),#2138,.T.);
#24385=ADVANCED_FACE('',(#3393),#2139,.T.);
#24386=ADVANCED_FACE('',(#3394),#2140,.T.);
#24387=ADVANCED_FACE('',(#3395),#2014,.T.);
#24388=ADVANCED_FACE('',(#3396),#2015,.T.);
#24389=ADVANCED_FACE('',(#3397),#2016,.T.);
#24390=ADVANCED_FACE('',(#3398),#2017,.T.);
#24391=ADVANCED_FACE('',(#3399),#2018,.T.);
#24392=ADVANCED_FACE('',(#3400),#2019,.T.);
#24393=ADVANCED_FACE('',(#3401,#1317),#2020,.F.);
#24552=CLOSED_SHELL('',(#24353,#24354,#24355,#24356,#24357,#24358,#24359,
#24360,#24361,#24362,#24363,#24364,#24365,#24366,#24367,#24368,#24369,#24370,
#24371,#24372,#24373,#24374,#24375,#24376,#24377,#24378,#24379,#24380,#24381,
#24382,#24383,#24384,#24385,#24386,#24387,#24388,#24389,#24390,#24391,#24392,
#24393));
#27107=AXIS2_PLACEMENT_3D('',#56059,#33673,#33674);
#27108=AXIS2_PLACEMENT_3D('',#56060,#33675,#33676);
#27109=AXIS2_PLACEMENT_3D('',#56062,#33677,#33678);
#27110=AXIS2_PLACEMENT_3D('',#56064,#33679,#33680);
#27111=AXIS2_PLACEMENT_3D('',#56065,#33681,#33682);
#27112=AXIS2_PLACEMENT_3D('',#56094,#33683,#33684);
#27113=AXIS2_PLACEMENT_3D('',#56095,#33685,#33686);
#27114=AXIS2_PLACEMENT_3D('',#56096,#33687,#33688);
#27115=AXIS2_PLACEMENT_3D('',#56099,#33690,#33691);
#27116=AXIS2_PLACEMENT_3D('',#56100,#33692,#33693);
#27117=AXIS2_PLACEMENT_3D('',#56102,#33694,#33695);
#27118=AXIS2_PLACEMENT_3D('',#56103,#33696,#33697);
#27119=AXIS2_PLACEMENT_3D('',#56106,#33698,#33699);
#27120=AXIS2_PLACEMENT_3D('',#56114,#33700,#33701);
#27121=AXIS2_PLACEMENT_3D('',#56117,#33702,#33703);
#27122=AXIS2_PLACEMENT_3D('',#56125,#33704,#33705);
#27123=AXIS2_PLACEMENT_3D('',#56128,#33706,#33707);
#27124=AXIS2_PLACEMENT_3D('',#56142,#33709,#33710);
#27125=AXIS2_PLACEMENT_3D('',#56153,#33711,#33712);
#27126=AXIS2_PLACEMENT_3D('',#56155,#33713,#33714);
#27127=AXIS2_PLACEMENT_3D('',#56157,#33715,#33716);
#27128=AXIS2_PLACEMENT_3D('',#56158,#33717,#33718);
#27129=AXIS2_PLACEMENT_3D('',#56162,#33720,#33721);
#27130=AXIS2_PLACEMENT_3D('',#56164,#33722,#33723);
#27131=AXIS2_PLACEMENT_3D('',#56166,#33724,#33725);
#27132=AXIS2_PLACEMENT_3D('',#56168,#33726,#33727);
#27133=AXIS2_PLACEMENT_3D('',#56170,#33728,#33729);
#27134=AXIS2_PLACEMENT_3D('',#56171,#33730,#33731);
#27135=AXIS2_PLACEMENT_3D('',#56172,#33732,#33733);
#27136=AXIS2_PLACEMENT_3D('',#56174,#33734,#33735);
#27137=AXIS2_PLACEMENT_3D('',#56175,#33736,#33737);
#27138=AXIS2_PLACEMENT_3D('',#56177,#33738,#33739);
#27139=AXIS2_PLACEMENT_3D('',#56179,#33740,#33741);
#27140=AXIS2_PLACEMENT_3D('',#56181,#33742,#33743);
#27141=AXIS2_PLACEMENT_3D('',#56183,#33744,#33745);
#27142=AXIS2_PLACEMENT_3D('',#56184,#33746,#33747);
#27143=AXIS2_PLACEMENT_3D('',#56185,#33748,#33749);
#27144=AXIS2_PLACEMENT_3D('',#56187,#33750,#33751);
#27145=AXIS2_PLACEMENT_3D('',#56189,#33752,#33753);
#27146=AXIS2_PLACEMENT_3D('',#56191,#33754,#33755);
#27147=AXIS2_PLACEMENT_3D('',#56193,#33756,#33757);
#27148=AXIS2_PLACEMENT_3D('',#56194,#33758,#33759);
#27149=AXIS2_PLACEMENT_3D('',#56195,#33760,#33761);
#27150=AXIS2_PLACEMENT_3D('',#56199,#33764,#33765);
#27151=AXIS2_PLACEMENT_3D('',#56203,#33768,#33769);
#27152=AXIS2_PLACEMENT_3D('',#56207,#33772,#33773);
#27153=AXIS2_PLACEMENT_3D('',#56211,#33776,#33777);
#27154=AXIS2_PLACEMENT_3D('',#56215,#33780,#33781);
#27155=AXIS2_PLACEMENT_3D('',#56219,#33784,#33785);
#27156=AXIS2_PLACEMENT_3D('',#56225,#33789,#33790);
#27157=AXIS2_PLACEMENT_3D('',#56229,#33793,#33794);
#27158=AXIS2_PLACEMENT_3D('',#56233,#33797,#33798);
#27159=AXIS2_PLACEMENT_3D('',#56237,#33801,#33802);
#27160=AXIS2_PLACEMENT_3D('',#56241,#33805,#33806);
#27161=AXIS2_PLACEMENT_3D('',#56243,#33808,#33809);
#27162=AXIS2_PLACEMENT_3D('',#56244,#33810,#33811);
#27163=AXIS2_PLACEMENT_3D('',#56252,#33812,#33813);
#27164=AXIS2_PLACEMENT_3D('',#56260,#33814,#33815);
#27165=AXIS2_PLACEMENT_3D('',#56268,#33816,#33817);
#27166=AXIS2_PLACEMENT_3D('',#56276,#33818,#33819);
#27167=AXIS2_PLACEMENT_3D('',#56284,#33820,#33821);
#27168=AXIS2_PLACEMENT_3D('',#56292,#33822,#33823);
#27169=AXIS2_PLACEMENT_3D('',#56300,#33824,#33825);
#27170=AXIS2_PLACEMENT_3D('',#56308,#33826,#33827);
#27171=AXIS2_PLACEMENT_3D('',#56316,#33828,#33829);
#27172=AXIS2_PLACEMENT_3D('',#56324,#33830,#33831);
#27173=AXIS2_PLACEMENT_3D('',#56327,#33834,#33835);
#27174=AXIS2_PLACEMENT_3D('',#56329,#33837,#33838);
#27175=AXIS2_PLACEMENT_3D('',#56331,#33840,#33841);
#27176=AXIS2_PLACEMENT_3D('',#56333,#33843,#33844);
#27177=AXIS2_PLACEMENT_3D('',#56335,#33846,#33847);
#27178=AXIS2_PLACEMENT_3D('',#56336,#33848,#33849);
#33673=DIRECTION('axis',(0.,0.,1.));
#33674=DIRECTION('refdir',(1.,0.,0.));
#33675=DIRECTION('center_axis',(-6.99485272571294E-17,-0.923879532511288,
0.382683432365087));
#33676=DIRECTION('ref_axis',(0.,-0.382683432365087,-0.923879532511288));
#33677=DIRECTION('center_axis',(0.,0.923879532511288,-0.382683432365087));
#33678=DIRECTION('ref_axis',(0.,0.382683432365087,0.923879532511288));
#33679=DIRECTION('center_axis',(1.,-1.77588086089071E-17,1.39910753728411E-16));
#33680=DIRECTION('ref_axis',(-1.22464679914735E-16,0.382683432365087,0.923879532511288));
#33681=DIRECTION('center_axis',(-6.99485272571294E-17,-0.923879532511288,
0.382683432365087));
#33682=DIRECTION('ref_axis',(6.87413134363318E-33,-0.382683432365087,-0.923879532511288));
#33683=DIRECTION('center_axis',(-1.,1.77588086089071E-17,-1.39910753728411E-16));
#33684=DIRECTION('ref_axis',(-1.22464679914735E-16,0.382683432365087,0.923879532511288));
#33685=DIRECTION('center_axis',(-6.99485272571294E-17,-0.923879532511288,
0.382683432365087));
#33686=DIRECTION('ref_axis',(1.30371071656723E-32,-0.382683432365087,-0.923879532511288));
#33687=DIRECTION('center_axis',(-6.99485272571294E-17,-0.923879532511288,
0.382683432365087));
#33688=DIRECTION('ref_axis',(7.11155521594025E-34,-0.382683432365087,-0.923879532511288));
#33689=DIRECTION('',(1.0961176199419E-16,0.722104291896042,-0.691784208858019));
#33690=DIRECTION('center_axis',(-6.99485272571294E-17,-0.923879532511288,
0.382683432365087));
#33691=DIRECTION('ref_axis',(7.11155521594025E-34,-0.382683432365087,-0.923879532511288));
#33692=DIRECTION('center_axis',(-0.5,-0.33141357403559,-0.800103145191267));
#33693=DIRECTION('ref_axis',(-0.866025403784439,0.191341716182545,0.461939766255643));
#33694=DIRECTION('center_axis',(-6.99485272571294E-17,-0.923879532511288,
0.382683432365087));
#33695=DIRECTION('ref_axis',(-4.26190864642653E-32,-0.382683432365087,-0.923879532511288));
#33696=DIRECTION('center_axis',(0.,-0.923879532511288,0.382683432365087));
#33697=DIRECTION('ref_axis',(0.,-0.382683432365087,-0.923879532511288));
#33698=DIRECTION('center_axis',(0.,-0.923879532511288,0.382683432365087));
#33699=DIRECTION('ref_axis',(0.,-0.382683432365087,-0.923879532511288));
#33700=DIRECTION('center_axis',(0.,0.923879532511288,-0.382683432365087));
#33701=DIRECTION('ref_axis',(0.,0.382683432365087,0.923879532511288));
#33702=DIRECTION('center_axis',(0.,0.923879532511288,-0.382683432365087));
#33703=DIRECTION('ref_axis',(0.,0.382683432365087,0.923879532511288));
#33704=DIRECTION('center_axis',(0.,-0.923879532511288,0.382683432365087));
#33705=DIRECTION('ref_axis',(0.,-0.382683432365087,-0.923879532511288));
#33706=DIRECTION('center_axis',(0.,-0.923879532511288,0.382683432365087));
#33707=DIRECTION('ref_axis',(0.,-0.382683432365087,-0.923879532511288));
#33708=DIRECTION('',(0.,0.923879532511288,-0.382683432365087));
#33709=DIRECTION('center_axis',(0.,-0.923879532511288,0.382683432365087));
#33710=DIRECTION('ref_axis',(0.,-0.382683432365087,-0.923879532511288));
#33711=DIRECTION('center_axis',(0.,0.,-1.));
#33712=DIRECTION('ref_axis',(-1.,0.,0.));
#33713=DIRECTION('center_axis',(0.,0.,-1.));
#33714=DIRECTION('ref_axis',(-1.,0.,0.));
#33715=DIRECTION('center_axis',(0.,0.,-1.));
#33716=DIRECTION('ref_axis',(-1.,0.,0.));
#33717=DIRECTION('center_axis',(0.,0.,-1.));
#33718=DIRECTION('ref_axis',(-1.,0.,0.));
#33719=DIRECTION('',(0.,0.,1.));
#33720=DIRECTION('center_axis',(0.,0.,-1.));
#33721=DIRECTION('ref_axis',(-1.,0.,0.));
#33722=DIRECTION('center_axis',(0.,0.,-1.));
#33723=DIRECTION('ref_axis',(-1.,0.,0.));
#33724=DIRECTION('center_axis',(0.,0.,-1.));
#33725=DIRECTION('ref_axis',(-1.,0.,0.));
#33726=DIRECTION('center_axis',(0.,0.,-1.));
#33727=DIRECTION('ref_axis',(-1.,0.,0.));
#33728=DIRECTION('center_axis',(0.,0.,-1.));
#33729=DIRECTION('ref_axis',(-1.,0.,0.));
#33730=DIRECTION('center_axis',(0.,0.,-1.));
#33731=DIRECTION('ref_axis',(-1.,0.,0.));
#33732=DIRECTION('center_axis',(6.12323399573677E-17,0.,1.));
#33733=DIRECTION('ref_axis',(1.,0.,0.));
#33734=DIRECTION('center_axis',(1.22464679914735E-16,-1.,0.));
#33735=DIRECTION('ref_axis',(-1.,-1.22464679914735E-16,0.));
#33736=DIRECTION('center_axis',(0.,-0.923879532511288,0.382683432365087));
#33737=DIRECTION('ref_axis',(0.,-0.382683432365087,-0.923879532511288));
#33738=DIRECTION('center_axis',(0.,-0.923879532511288,0.382683432365087));
#33739=DIRECTION('ref_axis',(0.,-0.382683432365087,-0.923879532511288));
#33740=DIRECTION('center_axis',(0.,-0.923879532511288,0.382683432365087));
#33741=DIRECTION('ref_axis',(0.,-0.382683432365087,-0.923879532511288));
#33742=DIRECTION('center_axis',(0.,-0.923879532511288,0.382683432365087));
#33743=DIRECTION('ref_axis',(0.,-0.382683432365087,-0.923879532511288));
#33744=DIRECTION('center_axis',(0.,-0.923879532511288,0.382683432365087));
#33745=DIRECTION('ref_axis',(0.,-0.382683432365087,-0.923879532511288));
#33746=DIRECTION('center_axis',(0.,-0.923879532511288,0.382683432365087));
#33747=DIRECTION('ref_axis',(0.,-0.382683432365087,-0.923879532511288));
#33748=DIRECTION('center_axis',(0.,0.923879532511288,-0.382683432365087));
#33749=DIRECTION('ref_axis',(0.,0.382683432365087,0.923879532511288));
#33750=DIRECTION('center_axis',(0.,0.923879532511288,-0.382683432365087));
#33751=DIRECTION('ref_axis',(0.,0.382683432365087,0.923879532511288));
#33752=DIRECTION('center_axis',(0.,0.923879532511288,-0.382683432365087));
#33753=DIRECTION('ref_axis',(0.,0.382683432365087,0.923879532511288));
#33754=DIRECTION('center_axis',(0.,0.923879532511288,-0.382683432365087));
#33755=DIRECTION('ref_axis',(0.,0.382683432365087,0.923879532511288));
#33756=DIRECTION('center_axis',(0.,0.923879532511288,-0.382683432365087));
#33757=DIRECTION('ref_axis',(0.,0.382683432365087,0.923879532511288));
#33758=DIRECTION('center_axis',(0.,-0.923879532511288,0.382683432365087));
#33759=DIRECTION('ref_axis',(0.,-0.382683432365087,-0.923879532511288));
#33760=DIRECTION('center_axis',(0.,0.,1.));
#33761=DIRECTION('ref_axis',(1.,0.,0.));
#33762=DIRECTION('',(3.56799717200074E-15,-1.,0.));
#33763=DIRECTION('',(-0.866025403784438,-0.500000000000001,0.));
#33764=DIRECTION('center_axis',(0.,0.,1.));
#33765=DIRECTION('ref_axis',(1.,0.,0.));
#33766=DIRECTION('',(-0.866025403784438,-0.500000000000001,0.));
#33767=DIRECTION('',(-0.866025403784441,0.499999999999995,0.));
#33768=DIRECTION('center_axis',(0.,0.,1.));
#33769=DIRECTION('ref_axis',(1.,0.,0.));
#33770=DIRECTION('',(-0.866025403784441,0.499999999999995,0.));
#33771=DIRECTION('',(-1.05162021911601E-14,1.,0.));
#33772=DIRECTION('center_axis',(0.,0.,1.));
#33773=DIRECTION('ref_axis',(1.,0.,0.));
#33774=DIRECTION('',(-1.05162021911601E-14,1.,0.));
#33775=DIRECTION('',(0.866025403784434,0.500000000000007,0.));
#33776=DIRECTION('center_axis',(0.,0.,1.));
#33777=DIRECTION('ref_axis',(1.,0.,0.));
#33778=DIRECTION('',(0.866025403784434,0.500000000000007,0.));
#33779=DIRECTION('',(0.866025403784441,-0.499999999999995,0.));
#33780=DIRECTION('center_axis',(0.,0.,1.));
#33781=DIRECTION('ref_axis',(1.,0.,0.));
#33782=DIRECTION('',(0.866025403784441,-0.499999999999995,0.));
#33783=DIRECTION('',(3.56799717200074E-15,-1.,0.));
#33784=DIRECTION('center_axis',(0.499999999999995,0.866025403784442,0.));
#33785=DIRECTION('ref_axis',(-0.866025403784441,0.499999999999995,0.));
#33786=DIRECTION('',(-0.866025403784441,0.499999999999995,0.));
#33787=DIRECTION('',(0.,0.,1.));
#33788=DIRECTION('',(0.,0.,1.));
#33789=DIRECTION('center_axis',(1.,1.05162021911601E-14,0.));
#33790=DIRECTION('ref_axis',(-1.05162021911601E-14,1.,0.));
#33791=DIRECTION('',(-1.05162021911601E-14,1.,0.));
#33792=DIRECTION('',(0.,0.,1.));
#33793=DIRECTION('center_axis',(0.500000000000007,-0.866025403784435,0.));
#33794=DIRECTION('ref_axis',(0.866025403784435,0.500000000000007,0.));
#33795=DIRECTION('',(0.866025403784434,0.500000000000007,0.));
#33796=DIRECTION('',(0.,0.,1.));
#33797=DIRECTION('center_axis',(-0.499999999999995,-0.866025403784441,0.));
#33798=DIRECTION('ref_axis',(0.866025403784442,-0.499999999999995,0.));
#33799=DIRECTION('',(0.866025403784441,-0.499999999999995,0.));
#33800=DIRECTION('',(0.,0.,1.));
#33801=DIRECTION('center_axis',(-1.,-3.56799717200074E-15,0.));
#33802=DIRECTION('ref_axis',(3.56799717200074E-15,-1.,0.));
#33803=DIRECTION('',(3.56799717200074E-15,-1.,0.));
#33804=DIRECTION('',(0.,0.,1.));
#33805=DIRECTION('center_axis',(-0.500000000000001,0.866025403784438,0.));
#33806=DIRECTION('ref_axis',(-0.866025403784438,-0.500000000000001,0.));
#33807=DIRECTION('',(-0.866025403784438,-0.500000000000001,0.));
#33808=DIRECTION('center_axis',(0.,0.,1.));
#33809=DIRECTION('ref_axis',(1.,0.,0.));
#33810=DIRECTION('center_axis',(0.,0.923879532511288,-0.382683432365087));
#33811=DIRECTION('ref_axis',(0.,0.382683432365087,0.923879532511288));
#33812=DIRECTION('center_axis',(0.,0.923879532511288,-0.382683432365087));
#33813=DIRECTION('ref_axis',(0.,0.382683432365087,0.923879532511288));
#33814=DIRECTION('center_axis',(0.,0.923879532511288,-0.382683432365087));
#33815=DIRECTION('ref_axis',(1.22464679914735E-16,-0.382683432365087,-0.923879532511288));
#33816=DIRECTION('center_axis',(0.,0.923879532511288,-0.382683432365087));
#33817=DIRECTION('ref_axis',(0.,0.382683432365087,0.923879532511288));
#33818=DIRECTION('center_axis',(0.,0.923879532511288,-0.382683432365087));
#33819=DIRECTION('ref_axis',(0.,0.382683432365087,0.923879532511288));
#33820=DIRECTION('center_axis',(0.,-0.923879532511288,0.382683432365087));
#33821=DIRECTION('ref_axis',(0.,-0.382683432365087,-0.923879532511288));
#33822=DIRECTION('center_axis',(0.,-0.923879532511288,0.382683432365087));
#33823=DIRECTION('ref_axis',(0.,-0.382683432365087,-0.923879532511288));
#33824=DIRECTION('center_axis',(0.,-0.923879532511288,0.382683432365087));
#33825=DIRECTION('ref_axis',(-7.6571373978539E-16,0.382683432365087,0.923879532511288));
#33826=DIRECTION('center_axis',(0.,-0.923879532511288,0.382683432365087));
#33827=DIRECTION('ref_axis',(0.,-0.382683432365087,-0.923879532511288));
#33828=DIRECTION('center_axis',(0.,-0.923879532511288,0.382683432365087));
#33829=DIRECTION('ref_axis',(0.,-0.382683432365087,-0.923879532511288));
#33830=DIRECTION('center_axis',(-0.5,-0.331413574035589,-0.800103145191266));
#33831=DIRECTION('ref_axis',(-0.84802901144343,6.89411318440465E-18,0.529949804934655));
#33832=DIRECTION('',(0.,0.923879532511288,-0.382683432365087));
#33833=DIRECTION('',(0.,0.923879532511288,-0.382683432365087));
#33834=DIRECTION('center_axis',(-1.,4.14906208744436E-17,1.00167219626363E-16));
#33835=DIRECTION('ref_axis',(1.00167219626363E-16,0.,1.));
#33836=DIRECTION('',(0.,0.923879532511288,-0.382683432365087));
#33837=DIRECTION('center_axis',(-0.5,0.331413574035589,0.800103145191267));
#33838=DIRECTION('ref_axis',(0.848029011443431,-1.03411697766071E-17,0.529949804934654));
#33839=DIRECTION('',(0.,0.923879532511288,-0.382683432365087));
#33840=DIRECTION('center_axis',(0.5,0.331413574035589,0.800103145191267));
#33841=DIRECTION('ref_axis',(0.84802901144343,-3.44705659220234E-18,-0.529949804934655));
#33842=DIRECTION('',(0.,0.923879532511288,-0.382683432365087));
#33843=DIRECTION('center_axis',(1.,0.,0.));
#33844=DIRECTION('ref_axis',(0.,0.,-1.));
#33845=DIRECTION('',(0.,0.923879532511288,-0.382683432365087));
#33846=DIRECTION('center_axis',(0.499999999999999,-0.33141357403559,-0.800103145191267));
#33847=DIRECTION('ref_axis',(-0.848029011443431,5.08102344929861E-18,-0.529949804934654));
#33848=DIRECTION('center_axis',(-6.99485272571294E-17,-0.923879532511288,
0.382683432365087));
#33849=DIRECTION('ref_axis',(-2.37033238942555E-33,-0.382683432365087,-0.923879532511288));
#56059=CARTESIAN_POINT('',(0.,0.,0.));
#56060=CARTESIAN_POINT('Origin',(-1.30104260698261E-15,5.62313017679403,
-9.43017678221748));
#56061=CARTESIAN_POINT('',(-9.42566476249075E-16,6.10854241414471,-5.90647463868609));
#56062=CARTESIAN_POINT('Origin',(-1.30104260698261E-15,4.79163859753386,
-9.0857616930889));
#56063=CARTESIAN_POINT('',(-1.65091236461116E-15,7.42947410803995,-6.70023456114395));
#56064=CARTESIAN_POINT('Origin',(-1.82151749662023E-15,7.24953476434565,
-5.50368876904451));
#56065=CARTESIAN_POINT('Origin',(-1.1944312217556E-15,6.1997608355023,-9.66902502153458));
#56066=CARTESIAN_POINT('Ctrl Pts',(-1.0334492107102E-15,9.1104629285565,
-7.23378761718564));
#56067=CARTESIAN_POINT('Ctrl Pts',(-3.36374346224613,9.1104629285565,-7.23378761718564));
#56068=CARTESIAN_POINT('Ctrl Pts',(-3.36374346224613,7.82321403482853,-10.3414813545735));
#56069=CARTESIAN_POINT('Ctrl Pts',(-3.36374346224613,6.53596514110056,-13.4491750919613));
#56070=CARTESIAN_POINT('Ctrl Pts',(-1.0334492107102E-15,6.53596514110056,
-13.4491750919613));
#56071=CARTESIAN_POINT('Ctrl Pts',(3.36374346224612,6.53596514110056,-13.4491750919613));
#56072=CARTESIAN_POINT('Ctrl Pts',(3.36374346224612,7.82321403482853,-10.3414813545735));
#56073=CARTESIAN_POINT('Ctrl Pts',(3.36374346224612,9.1104629285565,-7.23378761718564));
#56074=CARTESIAN_POINT('Ctrl Pts',(-1.0334492107102E-15,9.1104629285565,
-7.23378761718564));
#56075=CARTESIAN_POINT('Ctrl Pts',(-1.09748950322703E-15,8.40101827381132,
-6.55413148618164));
#56076=CARTESIAN_POINT('Ctrl Pts',(-3.72017113527558,8.40101827381132,-6.55413148618164));
#56077=CARTESIAN_POINT('Ctrl Pts',(-3.72017113527558,6.97737041477854,-9.99112145550203));
#56078=CARTESIAN_POINT('Ctrl Pts',(-3.72017113527558,5.55372255574576,-13.4281114248224));
#56079=CARTESIAN_POINT('Ctrl Pts',(-1.09748950322703E-15,5.55372255574576,
-13.4281114248224));
#56080=CARTESIAN_POINT('Ctrl Pts',(3.72017113527558,5.55372255574576,-13.4281114248224));
#56081=CARTESIAN_POINT('Ctrl Pts',(3.72017113527558,6.97737041477854,-9.99112145550203));
#56082=CARTESIAN_POINT('Ctrl Pts',(3.72017113527558,8.40101827381132,-6.55413148618164));
#56083=CARTESIAN_POINT('Ctrl Pts',(-1.09748950322703E-15,8.40101827381132,
-6.55413148618164));
#56084=CARTESIAN_POINT('Ctrl Pts',(-1.15636367776747E-15,7.42947410803995,
-6.70023456114395));
#56085=CARTESIAN_POINT('Ctrl Pts',(-3.21339563862928,7.42947410803995,-6.70023456114395));
#56086=CARTESIAN_POINT('Ctrl Pts',(-3.21339563862928,6.1997608355023,-9.66902502153458));
#56087=CARTESIAN_POINT('Ctrl Pts',(-3.21339563862928,4.97004756296464,-12.6378154819252));
#56088=CARTESIAN_POINT('Ctrl Pts',(-1.15636367776747E-15,4.97004756296464,
-12.6378154819252));
#56089=CARTESIAN_POINT('Ctrl Pts',(3.21339563862928,4.97004756296464,-12.6378154819252));
#56090=CARTESIAN_POINT('Ctrl Pts',(3.21339563862928,6.1997608355023,-9.66902502153458));
#56091=CARTESIAN_POINT('Ctrl Pts',(3.21339563862928,7.42947410803995,-6.70023456114395));
#56092=CARTESIAN_POINT('Ctrl Pts',(-1.15636367776747E-15,7.42947410803995,
-6.70023456114395));
#56093=CARTESIAN_POINT('',(-1.44538897712945E-15,9.1104629285565,-7.23378761718564));
#56094=CARTESIAN_POINT('Origin',(-1.26789919235761E-15,7.72689451084046,
-8.67799620097772));
#56095=CARTESIAN_POINT('Origin',(-1.07151675469833E-15,7.82321403482853,
-10.3414813545735));
#56096=CARTESIAN_POINT('Origin',(-9.16325707068394E-16,9.87297602634596,
-11.1905205710969));
#56097=CARTESIAN_POINT('',(-1.22248740685523E-15,10.8296846072587,-8.88082173981866));
#56098=CARTESIAN_POINT('',(-1.22248740685523E-15,10.8296846072587,-8.88082173981866));
#56099=CARTESIAN_POINT('Origin',(-9.16325707068394E-16,9.87297602634596,
-11.1905205710969));
#56100=CARTESIAN_POINT('Origin',(-8.67361737988404E-16,9.41103626009031,
-10.9991788549143));
#56101=CARTESIAN_POINT('',(0.944722181384557,9.66424685661039,-11.6944373635354));
#56102=CARTESIAN_POINT('Origin',(-9.16325707068394E-16,9.87297602634596,
-11.1905205710969));
#56103=CARTESIAN_POINT('Origin',(0.,4.50578927537974,-8.96735902705751));
#56104=CARTESIAN_POINT('',(-1.73205080756888,3.64358830043861,-11.8574002906228));
#56105=CARTESIAN_POINT('',(1.73205080756888,3.64358830043861,-11.8574002906228));
#56106=CARTESIAN_POINT('Origin',(0.,4.79163859753386,-9.08576169308891));
#56107=CARTESIAN_POINT('',(-8.67361737988404E-16,2.97505554591939,-12.6628771571027));
#56108=CARTESIAN_POINT('Ctrl Pts',(-8.83559534733916E-12,2.97505554591472,
-12.6628771571063));
#56109=CARTESIAN_POINT('Ctrl Pts',(0.928203230271955,3.46598430139072,-12.2861742738559));
#56110=CARTESIAN_POINT('Ctrl Pts',(1.73205080756887,3.6435883004386,-11.8574002906228));
#56111=CARTESIAN_POINT('Ctrl Pts',(-1.73205080756888,3.64358830043861,-11.8574002906228));
#56112=CARTESIAN_POINT('Ctrl Pts',(-0.928203230271849,3.46598430139071,
-12.2861742738559));
#56113=CARTESIAN_POINT('Ctrl Pts',(9.11080614203771E-12,2.97505554591457,
-12.6628771571064));
#56114=CARTESIAN_POINT('Origin',(0.,2.94387953251129,-8.32039482835873));
#56115=CARTESIAN_POINT('',(-1.73205080756888,4.09192982960656,-5.54875623082487));
#56116=CARTESIAN_POINT('',(1.73205080756888,4.09192982960656,-5.54875623082487));
#56117=CARTESIAN_POINT('Origin',(0.,2.94387953251129,-8.32039482835873));
#56118=CARTESIAN_POINT('',(6.50521303491303E-15,4.76046258412578,-4.74327936434497));
#56119=CARTESIAN_POINT('Ctrl Pts',(-8.84140945978337E-12,4.76046258413045,
-4.74327936434139));
#56120=CARTESIAN_POINT('Ctrl Pts',(0.928203230271958,4.26953382865444,-5.11998224759177));
#56121=CARTESIAN_POINT('Ctrl Pts',(1.73205080756888,4.09192982960656,-5.54875623082487));
#56122=CARTESIAN_POINT('Ctrl Pts',(-1.73205080756888,4.09192982960655,-5.54875623082487));
#56123=CARTESIAN_POINT('Ctrl Pts',(-0.928203230271845,4.26953382865446,
-5.11998224759171));
#56124=CARTESIAN_POINT('Ctrl Pts',(9.11907870314464E-12,4.7604625841306,
-4.74327936434127));
#56125=CARTESIAN_POINT('Origin',(0.,0.,-7.101));
#56126=CARTESIAN_POINT('',(-2.79266716119615,2.86374058300968,-7.101));
#56127=CARTESIAN_POINT('',(2.79266716119615,2.86374058300968,-7.101));
#56128=CARTESIAN_POINT('Origin',(0.,2.44435548440748,-8.11348519290263));
#56129=CARTESIAN_POINT('',(-4.61252776028392E-16,4.,-5.51067764861519));
#56130=CARTESIAN_POINT('Ctrl Pts',(-2.79266716119614,2.86374058300969,-7.10099999999999));
#56131=CARTESIAN_POINT('Ctrl Pts',(-2.791487395233,2.86489106908469,-7.0982224809144));
#56132=CARTESIAN_POINT('Ctrl Pts',(-2.79030270745925,2.86604495955758,-7.09544824938184));
#56133=CARTESIAN_POINT('Ctrl Pts',(-2.64444489381139,3.00792702197672,-6.75569806071638));
#56134=CARTESIAN_POINT('Ctrl Pts',(-2.42146694806281,3.19843151589414,-6.46722664985982));
#56135=CARTESIAN_POINT('Ctrl Pts',(-1.897815678339,3.53535819041829,-6.01625804314877));
#56136=CARTESIAN_POINT('Ctrl Pts',(-1.5580225174343,3.70511768616704,-5.82557882438308));
#56137=CARTESIAN_POINT('Ctrl Pts',(-0.804950314595278,3.93794187104499,
-5.57277579859251));
#56138=CARTESIAN_POINT('Ctrl Pts',(-0.391351836138015,4.,-5.51067764861519));
#56139=CARTESIAN_POINT('Ctrl Pts',(-3.46944695195361E-16,4.,-5.51067764861519));
#56140=CARTESIAN_POINT('',(-3.67394039744206E-16,4.09192982960655,-5.54875623082487));
#56141=CARTESIAN_POINT('',(-3.67394039744206E-16,1.14805029709526,-4.32936140246614));
#56142=CARTESIAN_POINT('Origin',(0.,2.94387953251129,-8.32039482835873));
#56143=CARTESIAN_POINT('Ctrl Pts',(-5.55111512312578E-16,4.,-5.51067764861519));
#56144=CARTESIAN_POINT('Ctrl Pts',(0.391351836138015,4.,-5.51067764861519));
#56145=CARTESIAN_POINT('Ctrl Pts',(0.804950314595278,3.93794187104499,-5.57277579859251));
#56146=CARTESIAN_POINT('Ctrl Pts',(1.5580225174343,3.70511768616704,-5.82557882438308));
#56147=CARTESIAN_POINT('Ctrl Pts',(1.897815678339,3.53535819041829,-6.01625804314877));
#56148=CARTESIAN_POINT('Ctrl Pts',(2.42146694806282,3.19843151589414,-6.46722664985983));
#56149=CARTESIAN_POINT('Ctrl Pts',(2.64444489381139,3.00792702197672,-6.75569806071639));
#56150=CARTESIAN_POINT('Ctrl Pts',(2.79030270745925,2.86604495955758,-7.09544824938184));
#56151=CARTESIAN_POINT('Ctrl Pts',(2.791487395233,2.86489106908469,-7.0982224809144));
#56152=CARTESIAN_POINT('Ctrl Pts',(2.79266716119614,2.86374058300969,-7.10099999999999));
#56153=CARTESIAN_POINT('Origin',(0.,0.,-13.5441803724939));
#56154=CARTESIAN_POINT('',(4.,-4.89858719658941E-16,-7.101));
#56155=CARTESIAN_POINT('Origin',(0.,0.,-7.101));
#56156=CARTESIAN_POINT('',(-4.,-4.89858719658941E-16,-7.101));
#56157=CARTESIAN_POINT('Origin',(0.,0.,-7.101));
#56158=CARTESIAN_POINT('Origin',(0.,0.,-7.101));
#56159=CARTESIAN_POINT('',(4.,4.20648087646404E-14,-3.));
#56160=CARTESIAN_POINT('',(4.,-4.89858719658941E-16,-13.5441803724939));
#56161=CARTESIAN_POINT('',(2.00000000000003,-3.46410161513774,-3.));
#56162=CARTESIAN_POINT('Origin',(0.,0.,-3.));
#56163=CARTESIAN_POINT('',(-1.99999999999998,-3.46410161513777,-3.));
#56164=CARTESIAN_POINT('Origin',(0.,0.,-3.));
#56165=CARTESIAN_POINT('',(-4.,-1.4271988688003E-14,-3.));
#56166=CARTESIAN_POINT('Origin',(0.,0.,-3.));
#56167=CARTESIAN_POINT('',(-2.,3.46410161513775,-3.));
#56168=CARTESIAN_POINT('Origin',(0.,0.,-3.));
#56169=CARTESIAN_POINT('',(1.99999999999999,3.46410161513778,-3.));
#56170=CARTESIAN_POINT('Origin',(0.,0.,-3.));
#56171=CARTESIAN_POINT('Origin',(0.,0.,-3.));
#56172=CARTESIAN_POINT('Origin',(0.,0.,-7.101));
#56173=CARTESIAN_POINT('',(-2.44929359829471E-16,-2.99951956532372E-32,
-11.101));
#56174=CARTESIAN_POINT('Origin',(0.,0.,-7.101));
#56175=CARTESIAN_POINT('Origin',(0.,6.32237232699421,-5.39024356304375));
#56176=CARTESIAN_POINT('',(3.46410161513776,4.79163859753387,-9.08576169308891));
#56177=CARTESIAN_POINT('Origin',(0.,4.79163859753387,-9.08576169308891));
#56178=CARTESIAN_POINT('',(-3.46410161513776,4.79163859753387,-9.08576169308891));
#56179=CARTESIAN_POINT('Origin',(0.,4.79163859753386,-9.08576169308891));
#56180=CARTESIAN_POINT('',(-1.73205080756888,5.93968889462913,-6.31412309555504));
#56181=CARTESIAN_POINT('Origin',(0.,4.79163859753386,-9.08576169308891));
#56182=CARTESIAN_POINT('',(1.73205080756888,5.93968889462913,-6.31412309555504));
#56183=CARTESIAN_POINT('Origin',(0.,4.79163859753386,-9.08576169308891));
#56184=CARTESIAN_POINT('Origin',(0.,4.79163859753386,-9.08576169308891));
#56185=CARTESIAN_POINT('Origin',(0.,4.47461326197163,-4.62487669831358));
#56186=CARTESIAN_POINT('',(3.46410161513776,2.94387953251129,-8.32039482835873));
#56187=CARTESIAN_POINT('Origin',(0.,2.94387953251129,-8.32039482835873));
#56188=CARTESIAN_POINT('',(-3.46410161513776,2.94387953251129,-8.32039482835873));
#56189=CARTESIAN_POINT('Origin',(0.,2.94387953251129,-8.32039482835873));
#56190=CARTESIAN_POINT('',(-1.73205080756888,1.79582923541603,-11.0920334258926));
#56191=CARTESIAN_POINT('Origin',(0.,2.94387953251129,-8.32039482835873));
#56192=CARTESIAN_POINT('',(1.73205080756888,1.79582923541603,-11.0920334258926));
#56193=CARTESIAN_POINT('Origin',(0.,2.94387953251129,-8.32039482835873));
#56194=CARTESIAN_POINT('Origin',(0.,2.94387953251129,-8.32039482835873));
#56195=CARTESIAN_POINT('Origin',(0.,0.,-3.));
#56196=CARTESIAN_POINT('',(-4.00000000000001,2.3094010767585,-3.));
#56197=CARTESIAN_POINT('',(-4.00000000000001,2.3094010767585,-3.));
#56198=CARTESIAN_POINT('',(0.,4.61880215351701,-3.));
#56199=CARTESIAN_POINT('Origin',(0.,0.,-3.));
#56200=CARTESIAN_POINT('',(0.,4.61880215351701,-3.));
#56201=CARTESIAN_POINT('',(0.,4.61880215351701,-3.));
#56202=CARTESIAN_POINT('',(3.99999999999998,2.30940107675855,-3.));
#56203=CARTESIAN_POINT('Origin',(0.,0.,-3.));
#56204=CARTESIAN_POINT('',(3.99999999999998,2.30940107675855,-3.));
#56205=CARTESIAN_POINT('',(3.99999999999998,2.30940107675855,-3.));
#56206=CARTESIAN_POINT('',(4.00000000000002,-2.30940107675847,-3.));
#56207=CARTESIAN_POINT('Origin',(0.,0.,-3.));
#56208=CARTESIAN_POINT('',(4.00000000000002,-2.30940107675847,-3.));
#56209=CARTESIAN_POINT('',(4.00000000000002,-2.30940107675847,-3.));
#56210=CARTESIAN_POINT('',(3.22529230536262E-14,-4.61880215351701,-3.));
#56211=CARTESIAN_POINT('Origin',(0.,0.,-3.));
#56212=CARTESIAN_POINT('',(3.22529230536262E-14,-4.61880215351701,-3.));
#56213=CARTESIAN_POINT('',(3.22529230536262E-14,-4.61880215351701,-3.));
#56214=CARTESIAN_POINT('',(-3.99999999999999,-2.30940107675852,-3.));
#56215=CARTESIAN_POINT('Origin',(0.,0.,-3.));
#56216=CARTESIAN_POINT('',(-3.99999999999999,-2.30940107675852,-3.));
#56217=CARTESIAN_POINT('',(-3.99999999999999,-2.30940107675852,-3.));
#56218=CARTESIAN_POINT('',(-4.00000000000001,2.3094010767585,-3.));
#56219=CARTESIAN_POINT('Origin',(3.99999999999998,2.30940107675855,-3.));
#56220=CARTESIAN_POINT('',(3.99999999999998,2.30940107675855,0.));
#56221=CARTESIAN_POINT('',(0.,4.61880215351701,0.));
#56222=CARTESIAN_POINT('',(3.99999999999998,2.30940107675855,0.));
#56223=CARTESIAN_POINT('',(3.99999999999998,2.30940107675855,-3.));
#56224=CARTESIAN_POINT('',(0.,4.61880215351701,-3.));
#56225=CARTESIAN_POINT('Origin',(4.00000000000002,-2.30940107675847,-3.));
#56226=CARTESIAN_POINT('',(4.00000000000002,-2.30940107675847,0.));
#56227=CARTESIAN_POINT('',(4.00000000000002,-2.30940107675847,0.));
#56228=CARTESIAN_POINT('',(4.00000000000002,-2.30940107675847,-3.));
#56229=CARTESIAN_POINT('Origin',(3.22529230536262E-14,-4.61880215351701,
-3.));
#56230=CARTESIAN_POINT('',(3.22529230536262E-14,-4.61880215351701,0.));
#56231=CARTESIAN_POINT('',(3.22529230536262E-14,-4.61880215351701,0.));
#56232=CARTESIAN_POINT('',(3.22529230536262E-14,-4.61880215351701,-3.));
#56233=CARTESIAN_POINT('Origin',(-3.99999999999999,-2.30940107675852,-3.));
#56234=CARTESIAN_POINT('',(-3.99999999999999,-2.30940107675852,0.));
#56235=CARTESIAN_POINT('',(-3.99999999999999,-2.30940107675852,0.));
#56236=CARTESIAN_POINT('',(-3.99999999999999,-2.30940107675852,-3.));
#56237=CARTESIAN_POINT('Origin',(-4.00000000000001,2.3094010767585,-3.));
#56238=CARTESIAN_POINT('',(-4.00000000000001,2.3094010767585,0.));
#56239=CARTESIAN_POINT('',(-4.00000000000001,2.3094010767585,0.));
#56240=CARTESIAN_POINT('',(-4.00000000000001,2.3094010767585,-3.));
#56241=CARTESIAN_POINT('Origin',(0.,4.61880215351701,-3.));
#56242=CARTESIAN_POINT('',(0.,4.61880215351701,0.));
#56243=CARTESIAN_POINT('Origin',(0.,0.,0.));
#56244=CARTESIAN_POINT('Origin',(0.,2.94387953251129,-8.32039482835873));
#56245=CARTESIAN_POINT('',(-3.46410161513776,3.9950957193956,-6.59103842936755));
#56246=CARTESIAN_POINT('Ctrl Pts',(-3.46410161513776,2.94387953251129,-8.32039482835873));
#56247=CARTESIAN_POINT('Ctrl Pts',(-3.46410161513776,3.29908753061063,-7.46284686188391));
#56248=CARTESIAN_POINT('Ctrl Pts',(-3.46410161513776,3.99509571941731,-6.59103842934036));
#56249=CARTESIAN_POINT('Ctrl Pts',(-3.46410161515884,3.99509571939744,-6.59103842938149));
#56250=CARTESIAN_POINT('Ctrl Pts',(-2.53589838487072,3.91432583055759,-5.97753021406059));
#56251=CARTESIAN_POINT('Ctrl Pts',(-1.73205080756888,4.09192982960655,-5.54875623082487));
#56252=CARTESIAN_POINT('Origin',(0.,2.94387953251129,-8.32039482835873));
#56253=CARTESIAN_POINT('',(-3.46410161513776,2.46436198993525,-10.2865565594127));
#56254=CARTESIAN_POINT('Ctrl Pts',(-1.73205080756888,1.79582923541603,-11.0920334258926));
#56255=CARTESIAN_POINT('Ctrl Pts',(-2.53589838486591,1.97343323446393,-10.6632594426594));
#56256=CARTESIAN_POINT('Ctrl Pts',(-3.46410161514687,2.46436198994007,-10.286556559409));
#56257=CARTESIAN_POINT('Ctrl Pts',(-3.46410161513776,2.46436198993072,-10.2865565594531));
#56258=CARTESIAN_POINT('Ctrl Pts',(-3.46410161513776,2.58867153441109,-9.17794279483566));
#56259=CARTESIAN_POINT('Ctrl Pts',(-3.46410161513776,2.94387953251129,-8.32039482835874));
#56260=CARTESIAN_POINT('Origin',(0.,2.94387953251129,-8.32039482835873));
#56261=CARTESIAN_POINT('',(3.90312782094782E-15,1.69899512520508,-12.1343156244353));
#56262=CARTESIAN_POINT('Ctrl Pts',(9.12142465330762E-12,1.69899512520587,
-12.1343156244413));
#56263=CARTESIAN_POINT('Ctrl Pts',(-0.928203230271842,1.61822523636812,
-11.5208074091258));
#56264=CARTESIAN_POINT('Ctrl Pts',(-1.73205080756888,1.79582923541603,-11.0920334258926));
#56265=CARTESIAN_POINT('Ctrl Pts',(1.73205080756888,1.79582923541603,-11.0920334258926));
#56266=CARTESIAN_POINT('Ctrl Pts',(0.928203230271956,1.61822523636815,-11.5208074091257));
#56267=CARTESIAN_POINT('Ctrl Pts',(-8.8435124366233E-12,1.69899512520584,
-12.1343156244411));
#56268=CARTESIAN_POINT('Origin',(0.,2.94387953251129,-8.32039482835873));
#56269=CARTESIAN_POINT('',(3.46410161513776,2.46436198993525,-10.2865565594127));
#56270=CARTESIAN_POINT('Ctrl Pts',(3.46410161514661,2.46436198993993,-10.2865565594091));
#56271=CARTESIAN_POINT('Ctrl Pts',(2.53589838486581,1.97343323446391,-10.6632594426595));
#56272=CARTESIAN_POINT('Ctrl Pts',(1.73205080756888,1.79582923541603,-11.0920334258926));
#56273=CARTESIAN_POINT('Ctrl Pts',(3.46410161513776,2.94387953251129,-8.32039482835873));
#56274=CARTESIAN_POINT('Ctrl Pts',(3.46410161513776,2.58867153441108,-9.17794279483565));
#56275=CARTESIAN_POINT('Ctrl Pts',(3.46410161513776,2.46436198993072,-10.2865565594531));
#56276=CARTESIAN_POINT('Origin',(0.,2.94387953251129,-8.32039482835873));
#56277=CARTESIAN_POINT('',(3.46410161513776,3.9950957193956,-6.59103842936756));
#56278=CARTESIAN_POINT('Ctrl Pts',(3.46410161513776,3.99509571941731,-6.59103842934036));
#56279=CARTESIAN_POINT('Ctrl Pts',(3.46410161513776,3.29908753061063,-7.46284686188391));
#56280=CARTESIAN_POINT('Ctrl Pts',(3.46410161513776,2.94387953251129,-8.32039482835873));
#56281=CARTESIAN_POINT('Ctrl Pts',(1.73205080756888,4.09192982960655,-5.54875623082487));
#56282=CARTESIAN_POINT('Ctrl Pts',(2.53589838487052,3.91432583055763,-5.97753021406048));
#56283=CARTESIAN_POINT('Ctrl Pts',(3.46410161515834,3.99509571939739,-6.59103842938115));
#56284=CARTESIAN_POINT('Origin',(0.,4.50578927537974,-8.96735902705751));
#56285=CARTESIAN_POINT('',(3.46410161513776,3.74042241064956,-10.8151180920801));
#56286=CARTESIAN_POINT('Ctrl Pts',(3.46410161513776,3.74042241062786,-10.8151180921073));
#56287=CARTESIAN_POINT('Ctrl Pts',(3.46410161513776,4.43643059943453,-9.94330965956373));
#56288=CARTESIAN_POINT('Ctrl Pts',(3.46410161513776,4.79163859753386,-9.08576169308893));
#56289=CARTESIAN_POINT('Ctrl Pts',(1.73205080756889,3.64358830043861,-11.8574002906228));
#56290=CARTESIAN_POINT('Ctrl Pts',(2.53589838487114,3.82119229948767,-11.4286263073868));
#56291=CARTESIAN_POINT('Ctrl Pts',(3.46410161515986,3.74042241064764,-10.8151180920655));
#56292=CARTESIAN_POINT('Origin',(0.,4.50578927537974,-8.96735902705751));
#56293=CARTESIAN_POINT('',(3.46410161513776,5.27115614010992,-7.11959996203494));
#56294=CARTESIAN_POINT('Ctrl Pts',(3.46410161514743,5.2711561401048,-7.11959996203886));
#56295=CARTESIAN_POINT('Ctrl Pts',(2.53589838486614,5.76208489558118,-6.74289707878832));
#56296=CARTESIAN_POINT('Ctrl Pts',(1.73205080756888,5.93968889462914,-6.31412309555504));
#56297=CARTESIAN_POINT('Ctrl Pts',(3.46410161513776,4.79163859753387,-9.08576169308891));
#56298=CARTESIAN_POINT('Ctrl Pts',(3.46410161513776,5.14684659563408,-8.22821372661199));
#56299=CARTESIAN_POINT('Ctrl Pts',(3.46410161513776,5.27115614011445,-7.11959996199452));
#56300=CARTESIAN_POINT('Origin',(0.,4.50578927537974,-8.96735902705751));
#56301=CARTESIAN_POINT('',(6.50521303491303E-15,6.03652300484009,-5.27184089701236));
#56302=CARTESIAN_POINT('Ctrl Pts',(9.66462909312592E-12,6.03652300483925,
-5.27184089700597));
#56303=CARTESIAN_POINT('Ctrl Pts',(-0.928203230271627,6.11729289367709,
-5.88534911232177));
#56304=CARTESIAN_POINT('Ctrl Pts',(-1.73205080756888,5.93968889462913,-6.31412309555505));
#56305=CARTESIAN_POINT('Ctrl Pts',(1.73205080756888,5.93968889462914,-6.31412309555504));
#56306=CARTESIAN_POINT('Ctrl Pts',(0.928203230271628,6.11729289367709,-5.88534911232177));
#56307=CARTESIAN_POINT('Ctrl Pts',(-9.6577405477995E-12,6.03652300483925,
-5.27184089700597));
#56308=CARTESIAN_POINT('Origin',(0.,4.50578927537974,-8.96735902705751));
#56309=CARTESIAN_POINT('',(-3.46410161513776,5.27115614010992,-7.11959996203493));
#56310=CARTESIAN_POINT('Ctrl Pts',(-3.46410161513776,5.27115614011445,-7.1195999619945));
#56311=CARTESIAN_POINT('Ctrl Pts',(-3.46410161513776,5.14684659563408,-8.22821372661199));
#56312=CARTESIAN_POINT('Ctrl Pts',(-3.46410161513776,4.79163859753387,-9.08576169308891));
#56313=CARTESIAN_POINT('Ctrl Pts',(-1.73205080756888,5.93968889462913,-6.31412309555505));
#56314=CARTESIAN_POINT('Ctrl Pts',(-2.53589838486613,5.76208489558118,-6.74289707878832));
#56315=CARTESIAN_POINT('Ctrl Pts',(-3.46410161514742,5.27115614010481,-7.11959996203885));
#56316=CARTESIAN_POINT('Origin',(0.,4.50578927537974,-8.96735902705751));
#56317=CARTESIAN_POINT('',(-3.46410161513776,3.74042241064957,-10.8151180920801));
#56318=CARTESIAN_POINT('Ctrl Pts',(-3.46410161515986,3.74042241064764,-10.8151180920655));
#56319=CARTESIAN_POINT('Ctrl Pts',(-2.53589838487113,3.82119229948767,-11.4286263073868));
#56320=CARTESIAN_POINT('Ctrl Pts',(-1.73205080756889,3.64358830043861,-11.8574002906228));
#56321=CARTESIAN_POINT('Ctrl Pts',(-3.46410161513776,4.79163859753387,-9.08576169308891));
#56322=CARTESIAN_POINT('Ctrl Pts',(-3.46410161513776,4.43643059943453,-9.94330965956373));
#56323=CARTESIAN_POINT('Ctrl Pts',(-3.46410161513776,3.74042241062786,-10.8151180921073));
#56324=CARTESIAN_POINT('Origin',(-8.67361737988404E-16,1.41314580305094,
-12.0159129584039));
#56325=CARTESIAN_POINT('',(-8.67361737988404E-16,1.41314580305094,-12.0159129584039));
#56326=CARTESIAN_POINT('',(-3.46410161513776,2.17851266778112,-10.1681538933813));
#56327=CARTESIAN_POINT('Origin',(-3.46410161513776,2.17851266778112,-10.1681538933813));
#56328=CARTESIAN_POINT('',(-3.46410161513776,3.70924639724147,-6.47263576333616));
#56329=CARTESIAN_POINT('Origin',(-3.46410161513776,3.70924639724147,-6.47263576333616));
#56330=CARTESIAN_POINT('',(7.02214595811131E-16,4.47461326197164,-4.62487669831358));
#56331=CARTESIAN_POINT('Origin',(7.02214595811131E-16,4.47461326197164,
-4.62487669831358));
#56332=CARTESIAN_POINT('',(3.46410161513776,3.70924639724147,-6.47263576333616));
#56333=CARTESIAN_POINT('Origin',(3.46410161513776,3.70924639724147,-6.47263576333616));
#56334=CARTESIAN_POINT('',(3.46410161513776,2.17851266778112,-10.1681538933813));
#56335=CARTESIAN_POINT('Origin',(3.46410161513776,2.17851266778112,-10.1681538933813));
#56336=CARTESIAN_POINT('Origin',(0.944722181384557,9.66424685661038,-11.6944373635354));
#57033=UNCERTAINTY_MEASURE_WITH_UNIT(LENGTH_MEASURE(0.01),#57080,
'DISTANCE_ACCURACY_VALUE',
'Maximum model space distance between geometric entities at asserted c
onnectivities');
#57040=UNCERTAINTY_MEASURE_WITH_UNIT(LENGTH_MEASURE(0.01),#57080,
'DISTANCE_ACCURACY_VALUE',
'Maximum model space distance between geometric entities at asserted c
onnectivities');
#57072=(
GEOMETRIC_REPRESENTATION_CONTEXT(3)
GLOBAL_UNCERTAINTY_ASSIGNED_CONTEXT((#57033))
GLOBAL_UNIT_ASSIGNED_CONTEXT((#57080,#57082,#57083))
REPRESENTATION_CONTEXT('','3D')
);
#57079=(
GEOMETRIC_REPRESENTATION_CONTEXT(3)
GLOBAL_UNCERTAINTY_ASSIGNED_CONTEXT((#57040))
GLOBAL_UNIT_ASSIGNED_CONTEXT((#57080,#57082,#57083))
REPRESENTATION_CONTEXT('','3D')
);
#57080=(
LENGTH_UNIT()
NAMED_UNIT(*)
SI_UNIT(.MILLI.,.METRE.)
);
#57082=(
NAMED_UNIT(*)
PLANE_ANGLE_UNIT()
SI_UNIT($,.RADIAN.)
);
#57083=(
NAMED_UNIT(*)
SI_UNIT($,.STERADIAN.)
SOLID_ANGLE_UNIT()
);
#57115=SHAPE_DEFINITION_REPRESENTATION(#57169,#57280);
#57169=PRODUCT_DEFINITION_SHAPE('',$,#57319);
#57280=SHAPE_REPRESENTATION('',(#27107),#57072);
#57287=PRODUCT_DEFINITION_CONTEXT('part definition',#57403,'design');
#57319=PRODUCT_DEFINITION('Slider End Cap','Slider End Cap',#57357,#57287);
#57357=PRODUCT_DEFINITION_FORMATION('',$,#57436);
#57403=APPLICATION_CONTEXT(
'Core Data for Automotive Mechanical Design Process');
#57404=PRODUCT_CONTEXT('part definition',#57403,'mechanical');
#57436=PRODUCT('Slider End Cap','Slider End Cap',$,(#57404));
#57444=PRESENTATION_STYLE_ASSIGNMENT((#57446));
#57446=SURFACE_STYLE_USAGE(.BOTH.,#57448);
#57448=SURFACE_SIDE_STYLE('',(#57450));
#57450=SURFACE_STYLE_FILL_AREA(#57452);
#57452=FILL_AREA_STYLE('Opaque(202,209,238)',(#57454));
#57454=FILL_AREA_STYLE_COLOUR('Opaque(202,209,238)',#57456);
#57456=COLOUR_RGB('Opaque(202,209,238)',0.792156862745098,0.819607843137255,
0.933333333333333);
ENDSEC;
END-ISO-10303-21;
